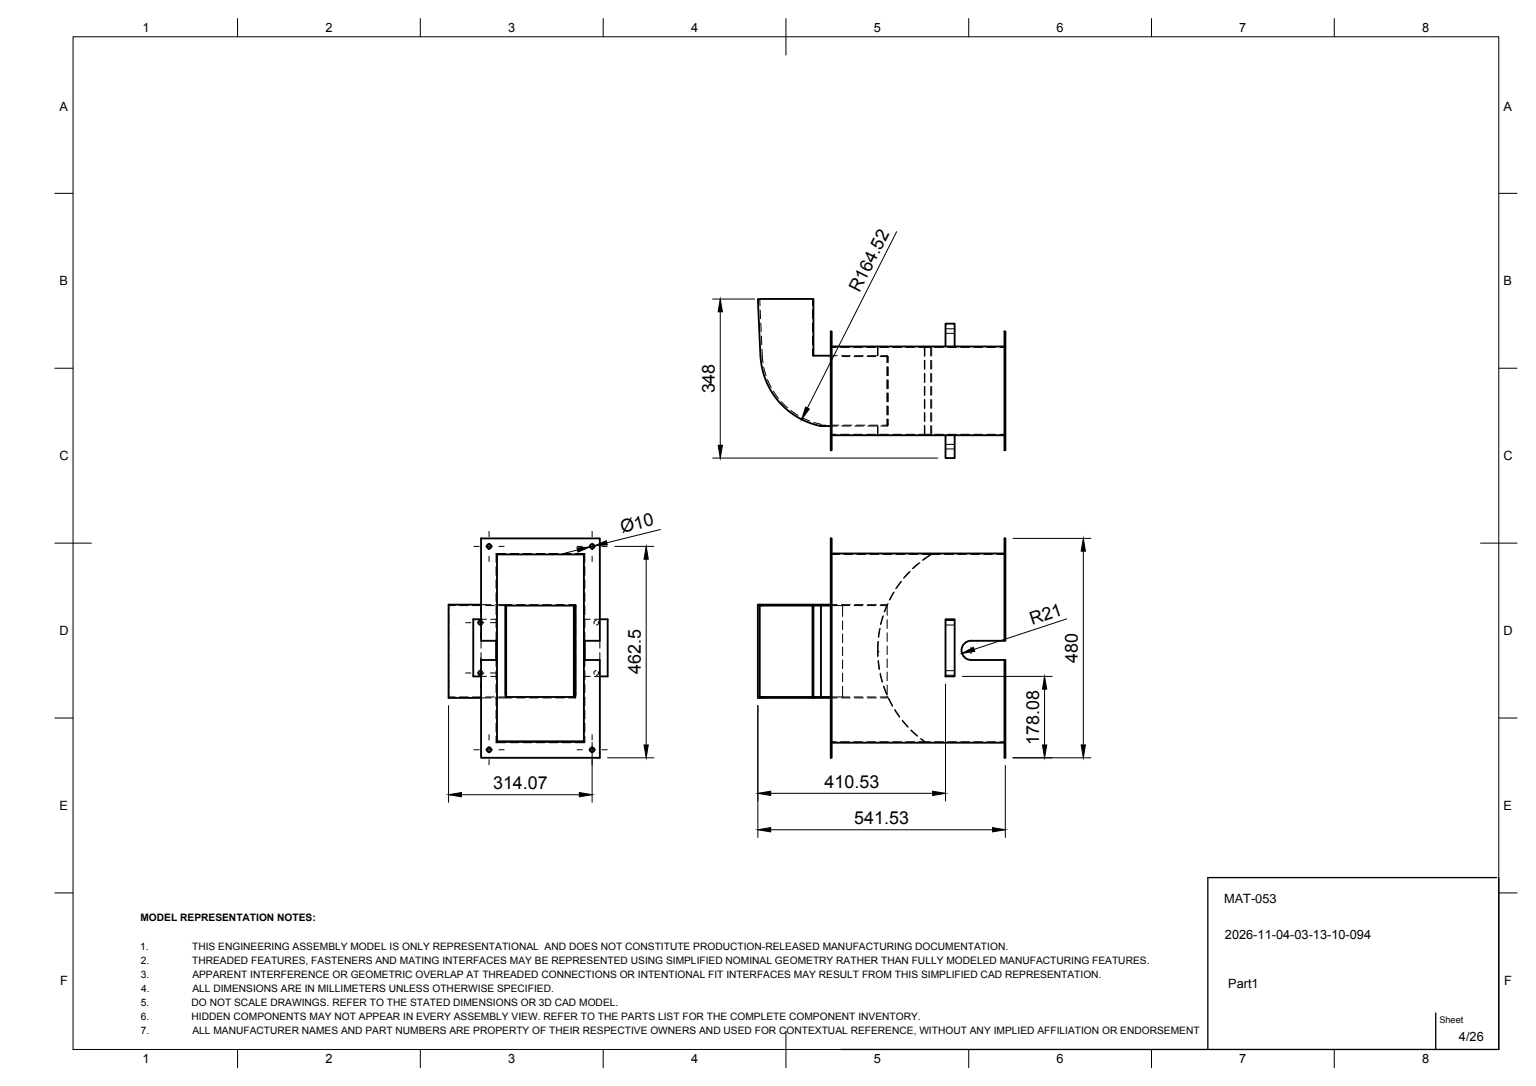
ISO-10303-21;
HEADER;
FILE_DESCRIPTION (('STEP AP214'),
    '1' );
FILE_NAME ('Part1.step',
    '2026-10-10T03:43:58',
    ( '' ),
    ( '' ),
    'SwSTEP 2.0',
    'SolidWorks 2026',
    '' );
FILE_SCHEMA (( 'AUTOMOTIVE_DESIGN' ));
ENDSEC;

DATA;
#9=VECTOR ( 'NONE', #58697, 1000.000000000000000 ) ;
#19=ORIENTED_EDGE ( 'NONE', *, *, #2654, .T. ) ;
#29=PLANE ( 'NONE',  #12068 ) ;
#34=AXIS2_PLACEMENT_3D ( 'NONE', #2299, #49415, #17054 ) ;
#77=DIRECTION ( 'NONE',  ( 1.000000000000000000, 0.000000000000000000, -0.000000000000000000 ) ) ;
#112=VECTOR ( 'NONE', #58293, 1000.000000000000000 ) ;
#116=DIRECTION ( 'NONE',  ( 0.000000000000000000, 0.000000000000000000, -1.000000000000000000 ) ) ;
#155=ORIENTED_EDGE ( 'NONE', *, *, #38259, .F. ) ;
#180=EDGE_LOOP ( 'NONE', ( #53944, #20596, #29884, #29507 ) ) ;
#185=LINE ( 'NONE', #21641, #40737 ) ;
#229=DIRECTION ( 'NONE',  ( 0.000000000000000000, 0.04541273895899431562, -0.9989683093773507050 ) ) ;
#230=EDGE_LOOP ( 'NONE', ( #67792, #13686 ) ) ;
#265=VECTOR ( 'NONE', #25443, 1000.000000000000000 ) ;
#289=ADVANCED_FACE ( 'NONE', ( #32988 ), #17141, .F. ) ;
#295=VERTEX_POINT ( 'NONE', #1681 ) ;
#297=EDGE_CURVE ( 'NONE', #67311, #11610, #65085, .T. ) ;
#314=EDGE_CURVE ( 'NONE', #536, #3478, #33702, .T. ) ;
#324=ORIENTED_EDGE ( 'NONE', *, *, #68515, .T. ) ;
#330=CARTESIAN_POINT ( 'NONE',  ( 444.9999999999999432, 225.0000000000000000, -2.000000000000000000 ) ) ;
#345=CARTESIAN_POINT ( 'NONE',  ( 0.000000000000000000, 0.000000000000000000, 380.0000000000000000 ) ) ;
#356=EDGE_CURVE ( 'NONE', #53205, #30991, #32306, .T. ) ;
#360=VECTOR ( 'NONE', #38064, 1000.000000000000000 ) ;
#401=ORIENTED_EDGE ( 'NONE', *, *, #69148, .T. ) ;
#408=ADVANCED_FACE ( 'NONE', ( #27013 ), #48440, .F. ) ;
#431=CARTESIAN_POINT ( 'NONE',  ( 111.9975424824652634, 296.0000000000000000, 529.9060149868646477 ) ) ;
#454=VERTEX_POINT ( 'NONE', #23494 ) ;
#463=EDGE_CURVE ( 'NONE', #12143, #43378, #39662, .T. ) ;
#473=EDGE_CURVE ( 'NONE', #23927, #8984, #16634, .T. ) ;
#477=ORIENTED_EDGE ( 'NONE', *, *, #56695, .T. ) ;
#491=ORIENTED_EDGE ( 'NONE', *, *, #35579, .F. ) ;
#527=DIRECTION ( 'NONE',  ( 0.000000000000000000, 0.000000000000000000, -1.000000000000000000 ) ) ;
#536=VERTEX_POINT ( 'NONE', #20279 ) ;
#575=ORIENTED_EDGE ( 'NONE', *, *, #1852, .T. ) ;
#606=VECTOR ( 'NONE', #8616, 1000.000000000000000 ) ;
#617=VECTOR ( 'NONE', #33046, 1000.000000000000000 ) ;
#626=VECTOR ( 'NONE', #27457, 1000.000000000000000 ) ;
#628=DIRECTION ( 'NONE',  ( -0.000000000000000000, -0.000000000000000000, -1.000000000000000000 ) ) ;
#653=ORIENTED_EDGE ( 'NONE', *, *, #46286, .F. ) ;
#654=EDGE_LOOP ( 'NONE', ( #13629, #60048, #33344, #59495 ) ) ;
#656=ORIENTED_EDGE ( 'NONE', *, *, #67416, .T. ) ;
#657=DIRECTION ( 'NONE',  ( 0.000000000000000000, -1.000000000000000000, 0.000000000000000000 ) ) ;
#675=DIRECTION ( 'NONE',  ( 0.000000000000000000, -1.000000000000000000, -0.000000000000000000 ) ) ;
#684=ORIENTED_EDGE ( 'NONE', *, *, #12471, .T. ) ;
#696=ORIENTED_EDGE ( 'NONE', *, *, #24415, .T. ) ;
#738=DIRECTION ( 'NONE',  ( -1.000000000000000000, 0.000000000000000000, 0.000000000000000000 ) ) ;
#821=DIRECTION ( 'NONE',  ( 0.000000000000000000, -0.000000000000000000, 1.000000000000000000 ) ) ;
#826=CYLINDRICAL_SURFACE ( 'NONE', #20311, 5.000000000000004441 ) ;
#992=LINE ( 'NONE', #5563, #37617 ) ;
#1020=EDGE_CURVE ( 'NONE', #49819, #55571, #66006, .T. ) ;
#1023=ORIENTED_EDGE ( 'NONE', *, *, #57399, .T. ) ;
#1033=CARTESIAN_POINT ( 'NONE',  ( 410.0000000000000000, -3.566368924055061292E-16, 174.3129005282752928 ) ) ;
#1037=ORIENTED_EDGE ( 'NONE', *, *, #10644, .F. ) ;
#1057=ORIENTED_EDGE ( 'NONE', *, *, #9172, .F. ) ;
#1060=FACE_OUTER_BOUND ( 'NONE', #18651, .T. ) ;
#1067=DIRECTION ( 'NONE',  ( 0.000000000000000000, 1.000000000000000000, 0.000000000000000000 ) ) ;
#1086=LINE ( 'NONE', #49961, #626 ) ;
#1118=CARTESIAN_POINT ( 'NONE',  ( 109.9975424824652634, 296.0000000000000000, 529.9060149868646477 ) ) ;
#1129=ORIENTED_EDGE ( 'NONE', *, *, #8619, .F. ) ;
#1165=DIRECTION ( 'NONE',  ( 0.000000000000000000, 0.000000000000000000, -1.000000000000000000 ) ) ;
#1188=EDGE_LOOP ( 'NONE', ( #37725, #12945, #49340, #52870, #24655, #3201, #47835, #3664 ) ) ;
#1198=VERTEX_POINT ( 'NONE', #53931 ) ;
#1228=ORIENTED_EDGE ( 'NONE', *, *, #39925, .F. ) ;
#1277=AXIS2_PLACEMENT_3D ( 'NONE', #30478, #35064, #25562 ) ;
#1357=DIRECTION ( 'NONE',  ( 0.000000000000000000, 0.000000000000000000, -1.000000000000000000 ) ) ;
#1379=DIRECTION ( 'NONE',  ( -0.000000000000000000, -0.000000000000000000, -1.000000000000000000 ) ) ;
#1399=ORIENTED_EDGE ( 'NONE', *, *, #17201, .T. ) ;
#1408=VERTEX_POINT ( 'NONE', #33562 ) ;
#1413=CARTESIAN_POINT ( 'NONE',  ( 209.9518228411288874, 0.000000000000000000, 31.43423095485942298 ) ) ;
#1424=PLANE ( 'NONE',  #7615 ) ;
#1458=DIRECTION ( 'NONE',  ( -1.000000000000000000, -0.000000000000000000, -0.000000000000000000 ) ) ;
#1464=ORIENTED_EDGE ( 'NONE', *, *, #14554, .T. ) ;
#1477=LINE ( 'NONE', #29259, #53207 ) ;
#1493=CARTESIAN_POINT ( 'NONE',  ( 410.0000000000000000, 0.000000000000000000, 380.0000000000000000 ) ) ;
#1496=ORIENTED_EDGE ( 'NONE', *, *, #11332, .F. ) ;
#1520=ORIENTED_EDGE ( 'NONE', *, *, #37790, .F. ) ;
#1535=VERTEX_POINT ( 'NONE', #23523 ) ;
#1558=EDGE_CURVE ( 'NONE', #28403, #51848, #17535, .T. ) ;
#1595=DIRECTION ( 'NONE',  ( 0.000000000000000000, 1.000000000000000000, 0.000000000000000000 ) ) ;
#1662=DIRECTION ( 'NONE',  ( -0.000000000000000000, -1.000000000000000000, -0.000000000000000000 ) ) ;
#1668=EDGE_CURVE ( 'NONE', #2382, #69500, #27304, .T. ) ;
#1680=VECTOR ( 'NONE', #34096, 1000.000000000000000 ) ;
#1681=CARTESIAN_POINT ( 'NONE',  ( 311.9975424824652350, 172.0000000000000284, 354.1673509436691347 ) ) ;
#1696=ORIENTED_EDGE ( 'NONE', *, *, #44720, .F. ) ;
#1705=ORIENTED_EDGE ( 'NONE', *, *, #28112, .T. ) ;
#1708=LINE ( 'NONE', #34768, #38008 ) ;
#1717=AXIS2_PLACEMENT_3D ( 'NONE', #66276, #45132, #30005 ) ;
#1732=CARTESIAN_POINT ( 'NONE',  ( 209.9999999999999716, 192.0000000000000000, 72.99999999999998579 ) ) ;
#1750=CARTESIAN_POINT ( 'NONE',  ( 432.4999999999999432, -18.06806526123148160, 378.0000000000000000 ) ) ;
#1783=AXIS2_PLACEMENT_3D ( 'NONE', #7114, #56339, #29267 ) ;
#1797=EDGE_LOOP ( 'NONE', ( #65731, #29293 ) ) ;
#1804=DIRECTION ( 'NONE',  ( 0.000000000000000000, -1.000000000000000000, 0.000000000000000000 ) ) ;
#1810=CARTESIAN_POINT ( 'NONE',  ( 0.000000000000000000, 190.0000000000000000, 159.3522585083728700 ) ) ;
#1812=CARTESIAN_POINT ( 'NONE',  ( 188.9999999999999432, 190.0000000000000000, 380.0000000000000000 ) ) ;
#1822=DIRECTION ( 'NONE',  ( -0.000000000000000000, -0.000000000000000000, -1.000000000000000000 ) ) ;
#1848=VECTOR ( 'NONE', #11811, 1000.000000000000000 ) ;
#1852=EDGE_CURVE ( 'NONE', #67175, #45635, #9379, .T. ) ;
#1854=CARTESIAN_POINT ( 'NONE',  ( -17.50000000000002842, -18.06806526123148160, 380.0000000000000000 ) ) ;
#1885=PLANE ( 'NONE',  #60224 ) ;
#1923=FACE_OUTER_BOUND ( 'NONE', #44162, .T. ) ;
#1974=PLANE ( 'NONE',  #39498 ) ;
#1986=LINE ( 'NONE', #30100, #9912 ) ;
#1987=CARTESIAN_POINT ( 'NONE',  ( 144.4165763529819344, -26.99999999999998224, 108.9999999999999858 ) ) ;
#2008=CARTESIAN_POINT ( 'NONE',  ( 313.9975424824652350, 172.0000000000000284, 418.0000000000000000 ) ) ;
#2012=CARTESIAN_POINT ( 'NONE',  ( 188.9999999999999432, 0.000000000000000000, 380.0000000000000000 ) ) ;
#2035=VECTOR ( 'NONE', #52358, 1000.000000000000000 ) ;
#2043=ORIENTED_EDGE ( 'NONE', *, *, #42498, .F. ) ;
#2047=CARTESIAN_POINT ( 'NONE',  ( 0.000000000000000000, 190.0000000000000000, -2.000000000000000000 ) ) ;
#2048=ORIENTED_EDGE ( 'NONE', *, *, #27631, .F. ) ;
#2063=CARTESIAN_POINT ( 'NONE',  ( 109.9975424824652634, 18.08738615523480675, 402.4289050101931480 ) ) ;
#2086=CIRCLE ( 'NONE', #66164, 246.3582898394606957 ) ;
#2097=DIRECTION ( 'NONE',  ( -1.000000000000000000, 0.000000000000000000, 0.000000000000000000 ) ) ;
#2105=ADVANCED_FACE ( 'NONE', ( #14188 ), #35648, .F. ) ;
#2115=CARTESIAN_POINT ( 'NONE',  ( 109.9975424824652634, 296.0000000000000000, 529.9060149868646477 ) ) ;
#2119=CARTESIAN_POINT ( 'NONE',  ( 309.8720357909272707, 172.0000000000000284, 536.6193948016162949 ) ) ;
#2126=VECTOR ( 'NONE', #628, 1000.000000000000000 ) ;
#2135=DIRECTION ( 'NONE',  ( 0.000000000000000000, 0.000000000000000000, 1.000000000000000000 ) ) ;
#2166=CARTESIAN_POINT ( 'NONE',  ( -12.50000000000002842, 207.5000000000000284, 378.0000000000000000 ) ) ;
#2179=DIRECTION ( 'NONE',  ( 0.000000000000000000, 0.000000000000000000, -1.000000000000000000 ) ) ;
#2210=VERTEX_POINT ( 'NONE', #64435 ) ;
#2229=AXIS2_PLACEMENT_3D ( 'NONE', #66577, #8161, #56011 ) ;
#2243=VERTEX_POINT ( 'NONE', #47217 ) ;
#2251=DIRECTION ( 'NONE',  ( 0.000000000000000000, 0.9989683093773507050, 0.04541273895899305274 ) ) ;
#2272=DIRECTION ( 'NONE',  ( 0.000000000000000000, 0.000000000000000000, 1.000000000000000000 ) ) ;
#2277=DIRECTION ( 'NONE',  ( -1.000000000000000000, 0.000000000000000000, 0.000000000000000000 ) ) ;
#2293=CARTESIAN_POINT ( 'NONE',  ( 427.4999999999999432, 207.5000000000000284, 0.000000000000000000 ) ) ;
#2299=CARTESIAN_POINT ( 'NONE',  ( 259.4165763529819060, 225.8585178651493948, 138.9999999999999716 ) ) ;
#2338=DIRECTION ( 'NONE',  ( 0.9216045519012663334, 0.000000000000000000, -0.3881301971180111110 ) ) ;
#2382=VERTEX_POINT ( 'NONE', #6028 ) ;
#2430=LINE ( 'NONE', #50964, #30805 ) ;
#2453=CARTESIAN_POINT ( 'NONE',  ( 0.000000000000000000, -2.000000000000000000, 380.0000000000000000 ) ) ;
#2507=LINE ( 'NONE', #49989, #5388 ) ;
#2535=FACE_OUTER_BOUND ( 'NONE', #48112, .T. ) ;
#2614=CARTESIAN_POINT ( 'NONE',  ( 264.4165763529819628, 225.8585178651493948, 128.9999999999999716 ) ) ;
#2626=VERTEX_POINT ( 'NONE', #43227 ) ;
#2641=AXIS2_PLACEMENT_3D ( 'NONE', #67736, #19535, #40994 ) ;
#2654=EDGE_CURVE ( 'NONE', #33368, #44925, #15052, .T. ) ;
#2674=ORIENTED_EDGE ( 'NONE', *, *, #30840, .F. ) ;
#2687=CARTESIAN_POINT ( 'NONE',  ( 111.9975424824652634, 0.000000000000000000, 256.6193948016162381 ) ) ;
#2727=ORIENTED_EDGE ( 'NONE', *, *, #23656, .F. ) ;
#2751=CARTESIAN_POINT ( 'NONE',  ( 444.9999999999999432, -35.00000000000000000, 380.0000000000000000 ) ) ;
#2809=CYLINDRICAL_SURFACE ( 'NONE', #65443, 245.3095347406802773 ) ;
#2815=DIRECTION ( 'NONE',  ( 1.000000000000000000, 0.000000000000000000, 0.000000000000000000 ) ) ;
#2816=PLANE ( 'NONE',  #19313 ) ;
#2821=DIRECTION ( 'NONE',  ( 0.000000000000000000, -1.000000000000000000, -0.000000000000000000 ) ) ;
#2831=AXIS2_PLACEMENT_3D ( 'NONE', #67732, #19884, #29741 ) ;
#2879=CARTESIAN_POINT ( 'NONE',  ( 432.4999999999999432, 207.5000000000000284, 0.000000000000000000 ) ) ;
#2887=VECTOR ( 'NONE', #14125, 1000.000000000000000 ) ;
#2902=ORIENTED_EDGE ( 'NONE', *, *, #54366, .F. ) ;
#2909=LINE ( 'NONE', #51449, #54074 ) ;
#2923=LINE ( 'NONE', #41930, #52350 ) ;
#2947=AXIS2_PLACEMENT_3D ( 'NONE', #10243, #42268, #36303 ) ;
#2957=VERTEX_POINT ( 'NONE', #32182 ) ;
#2963=LINE ( 'NONE', #57118, #66829 ) ;
#2974=DIRECTION ( 'NONE',  ( -1.000000000000000000, 0.000000000000000000, 0.000000000000000000 ) ) ;
#2986=LINE ( 'NONE', #66329, #33613 ) ;
#2999=AXIS2_PLACEMENT_3D ( 'NONE', #53087, #48837, #21109 ) ;
#3077=VECTOR ( 'NONE', #52022, 1000.000000000000000 ) ;
#3156=DIRECTION ( 'NONE',  ( -0.000000000000000000, 1.000000000000000000, -0.000000000000000000 ) ) ;
#3157=DIRECTION ( 'NONE',  ( 0.000000000000000000, 1.000000000000000000, 0.000000000000000000 ) ) ;
#3169=CARTESIAN_POINT ( 'NONE',  ( 213.7147529443549843, 172.0000000000000284, 277.7621479143228385 ) ) ;
#3182=ORIENTED_EDGE ( 'NONE', *, *, #20387, .F. ) ;
#3201=ORIENTED_EDGE ( 'NONE', *, *, #20529, .F. ) ;
#3202=DIRECTION ( 'NONE',  ( -1.000000000000000000, -0.000000000000000000, -0.000000000000000000 ) ) ;
#3213=ORIENTED_EDGE ( 'NONE', *, *, #23131, .T. ) ;
#3221=EDGE_LOOP ( 'NONE', ( #1037, #38280, #21637, #19798 ) ) ;
#3262=ORIENTED_EDGE ( 'NONE', *, *, #53398, .F. ) ;
#3263=EDGE_CURVE ( 'NONE', #46362, #11641, #10625, .T. ) ;
#3278=CARTESIAN_POINT ( 'NONE',  ( -17.50000000000002842, 207.5000000000000284, 380.0000000000000000 ) ) ;
#3313=LINE ( 'NONE', #24774, #4136 ) ;
#3315=ORIENTED_EDGE ( 'NONE', *, *, #43959, .F. ) ;
#3333=EDGE_CURVE ( 'NONE', #9171, #11778, #44252, .T. ) ;
#3363=FACE_OUTER_BOUND ( 'NONE', #61772, .T. ) ;
#3375=LINE ( 'NONE', #67747, #44396 ) ;
#3403=ORIENTED_EDGE ( 'NONE', *, *, #15348, .F. ) ;
#3425=DIRECTION ( 'NONE',  ( -0.8532989592251508659, 0.000000000000000000, 0.5214219847544543374 ) ) ;
#3463=CARTESIAN_POINT ( 'NONE',  ( 422.4999999999999432, 207.5000000000000284, -2.000000000000000000 ) ) ;
#3478=VERTEX_POINT ( 'NONE', #65860 ) ;
#3486=CARTESIAN_POINT ( 'NONE',  ( 209.9518228411288874, 18.00000000000002842, 31.43423095485942298 ) ) ;
#3498=EDGE_CURVE ( 'NONE', #14375, #1535, #61261, .T. ) ;
#3500=CARTESIAN_POINT ( 'NONE',  ( 149.4165763529819344, -26.99999999999998224, 108.9999999999999858 ) ) ;
#3521=CARTESIAN_POINT ( 'NONE',  ( -12.50000000000002842, -18.06806526123148160, 380.0000000000000000 ) ) ;
#3574=DIRECTION ( 'NONE',  ( 1.000000000000000000, 0.000000000000000000, -0.000000000000000000 ) ) ;
#3602=CARTESIAN_POINT ( 'NONE',  ( 427.4999999999999432, -18.06806526123148160, -2.000000000000000000 ) ) ;
#3604=DIRECTION ( 'NONE',  ( 2.220446049250313081E-16, 0.000000000000000000, 1.000000000000000000 ) ) ;
#3610=CYLINDRICAL_SURFACE ( 'NONE', #28683, 246.3582898394606957 ) ;
#3619=CARTESIAN_POINT ( 'NONE',  ( 444.9999999999999432, 225.0000000000000000, 0.000000000000000000 ) ) ;
#3653=FACE_BOUND ( 'NONE', #46999, .T. ) ;
#3654=DIRECTION ( 'NONE',  ( -1.000000000000000000, 0.000000000000000000, 0.000000000000000000 ) ) ;
#3659=ORIENTED_EDGE ( 'NONE', *, *, #14979, .F. ) ;
#3664=ORIENTED_EDGE ( 'NONE', *, *, #5871, .F. ) ;
#3673=( LENGTH_UNIT ( ) NAMED_UNIT ( * ) SI_UNIT ( .MILLI., .METRE. ) );
#3696=FACE_OUTER_BOUND ( 'NONE', #32892, .T. ) ;
#3707=ORIENTED_EDGE ( 'NONE', *, *, #60071, .F. ) ;
#3743=CARTESIAN_POINT ( 'NONE',  ( 149.4165763529819344, 225.8585178651493663, 108.9999999999999858 ) ) ;
#3750=DIRECTION ( 'NONE',  ( -1.000000000000000000, 0.000000000000000000, 0.000000000000000000 ) ) ;
#3790=EDGE_LOOP ( 'NONE', ( #19909, #52215, #66218, #50084 ) ) ;
#3813=EDGE_CURVE ( 'NONE', #2957, #57714, #49733, .T. ) ;
#3841=FACE_OUTER_BOUND ( 'NONE', #20050, .T. ) ;
#3843=EDGE_CURVE ( 'NONE', #35195, #22151, #28650, .T. ) ;
#3853=DIRECTION ( 'NONE',  ( -1.000000000000000000, 0.000000000000000000, 0.000000000000000000 ) ) ;
#3862=CYLINDRICAL_SURFACE ( 'NONE', #39982, 5.000000000000000888 ) ;
#3869=LINE ( 'NONE', #20730, #10810 ) ;
#3895=AXIS2_PLACEMENT_3D ( 'NONE', #1732, #33745, #7004 ) ;
#3933=VECTOR ( 'NONE', #53497, 1000.000000000000000 ) ;
#3945=LINE ( 'NONE', #57754, #60605 ) ;
#3947=CARTESIAN_POINT ( 'NONE',  ( 444.9999999999999432, -35.00000000000000000, -2.000000000000000000 ) ) ;
#3950=PRODUCT_DEFINITION ( 'UNKNOWN', '', #68169, #43669 ) ;
#3953=DIRECTION ( 'NONE',  ( 0.000000000000000000, 0.000000000000000000, -1.000000000000000000 ) ) ;
#3979=EDGE_LOOP ( 'NONE', ( #60158, #1057, #656, #3707 ) ) ;
#3987=AXIS2_PLACEMENT_3D ( 'NONE', #45053, #29926, #14093 ) ;
#3989=CYLINDRICAL_SURFACE ( 'NONE', #60363, 246.3582898394606957 ) ;
#4006=DIRECTION ( 'NONE',  ( -0.000000000000000000, -0.000000000000000000, 1.000000000000000000 ) ) ;
#4015=CARTESIAN_POINT ( 'NONE',  ( 444.9999999999999432, 225.0000000000000000, 380.0000000000000000 ) ) ;
#4018=FACE_BOUND ( 'NONE', #5277, .T. ) ;
#4026=SURFACE_SIDE_STYLE ('',( #64140 ) ) ;
#4032=DIRECTION ( 'NONE',  ( -0.000000000000000000, 1.000000000000000000, 0.000000000000000000 ) ) ;
#4136=VECTOR ( 'NONE', #3654, 1000.000000000000000 ) ;
#4195=EDGE_CURVE ( 'NONE', #14640, #7559, #37718, .T. ) ;
#4205=ORIENTED_EDGE ( 'NONE', *, *, #66591, .T. ) ;
#4227=CARTESIAN_POINT ( 'NONE',  ( 230.9999999999999432, -2.000000000000000000, 0.000000000000000000 ) ) ;
#4247=ORIENTED_EDGE ( 'NONE', *, *, #45253, .T. ) ;
#4253=VECTOR ( 'NONE', #53682, 1000.000000000000000 ) ;
#4264=LINE ( 'NONE', #35927, #67110 ) ;
#4296=DIRECTION ( 'NONE',  ( 0.000000000000000000, 0.000000000000000000, 1.000000000000000000 ) ) ;
#4321=ADVANCED_FACE ( 'NONE', ( #52442, #69302, #10552 ), #59082, .F. ) ;
#4333=DIRECTION ( 'NONE',  ( 0.000000000000000000, -0.000000000000000000, 1.000000000000000000 ) ) ;
#4372=EDGE_CURVE ( 'NONE', #11778, #9171, #17235, .T. ) ;
#4381=CARTESIAN_POINT ( 'NONE',  ( 230.9999999999999432, 225.0000000000000000, -2.000000000000000000 ) ) ;
#4410=AXIS2_PLACEMENT_3D ( 'NONE', #23079, #24730, #27991 ) ;
#4431=EDGE_LOOP ( 'NONE', ( #49238, #30176, #26418, #57787, #61721, #36911, #47133, #38510 ) ) ;
#4435=CARTESIAN_POINT ( 'NONE',  ( 209.3223706822284100, 18.00000000000002842, 31.44247402469554942 ) ) ;
#4438=ORIENTED_EDGE ( 'NONE', *, *, #56470, .T. ) ;
#4439=EDGE_CURVE ( 'NONE', #61512, #35195, #55470, .T. ) ;
#4442=CARTESIAN_POINT ( 'NONE',  ( 144.4165763529819344, -26.99999999999998224, 129.0000000000000000 ) ) ;
#4445=AXIS2_PLACEMENT_3D ( 'NONE', #32054, #54172, #26777 ) ;
#4461=ORIENTED_EDGE ( 'NONE', *, *, #65946, .F. ) ;
#4514=EDGE_LOOP ( 'NONE', ( #56246, #66798, #21095, #54977 ) ) ;
#4522=VERTEX_POINT ( 'NONE', #37906 ) ;
#4527=EDGE_CURVE ( 'NONE', #58159, #37433, #21720, .T. ) ;
#4540=AXIS2_PLACEMENT_3D ( 'NONE', #13314, #56207, #63225 ) ;
#4549=CARTESIAN_POINT ( 'NONE',  ( 422.4999999999999432, 207.5000000000000284, 378.0000000000000000 ) ) ;
#4559=CARTESIAN_POINT ( 'NONE',  ( 188.9999999999999432, 192.0000000000000000, 380.0000000000000000 ) ) ;
#4573=ORIENTED_EDGE ( 'NONE', *, *, #57997, .F. ) ;
#4597=VERTEX_POINT ( 'NONE', #11501 ) ;
#4647=ORIENTED_EDGE ( 'NONE', *, *, #18931, .F. ) ;
#4665=DIRECTION ( 'NONE',  ( -0.000000000000000000, -1.000000000000000000, -0.000000000000000000 ) ) ;
#4690=AXIS2_PLACEMENT_3D ( 'NONE', #10679, #63473, #25852 ) ;
#4716=ORIENTED_EDGE ( 'NONE', *, *, #57128, .F. ) ;
#4717=ORIENTED_EDGE ( 'NONE', *, *, #37321, .T. ) ;
#4729=PLANE ( 'NONE',  #13598 ) ;
#4777=FACE_BOUND ( 'NONE', #67741, .T. ) ;
#4797=ORIENTED_EDGE ( 'NONE', *, *, #48258, .F. ) ;
#4803=CARTESIAN_POINT ( 'NONE',  ( 311.9975424824652350, 0.000000000000000000, 254.5114349394235091 ) ) ;
#4874=DIRECTION ( 'NONE',  ( 0.000000000000000000, -1.000000000000000000, 0.000000000000000000 ) ) ;
#4875=AXIS2_PLACEMENT_3D ( 'NONE', #67150, #56217, #8033 ) ;
#4894=ORIENTED_EDGE ( 'NONE', *, *, #26906, .F. ) ;
#4899=DIRECTION ( 'NONE',  ( 0.01527021686369653929, 0.000000000000000000, 0.9998834034410890581 ) ) ;
#4947=CARTESIAN_POINT ( 'NONE',  ( -2.000000000000000000, 192.0000000000000000, 0.000000000000000000 ) ) ;
#4950=CARTESIAN_POINT ( 'NONE',  ( 0.000000000000000000, 190.0000000000000000, 380.0000000000000000 ) ) ;
#4992=ORIENTED_EDGE ( 'NONE', *, *, #9172, .T. ) ;
#4993=DIRECTION ( 'NONE',  ( 0.000000000000000000, -0.04541273895899431562, 0.9989683093773507050 ) ) ;
#5038=DIRECTION ( 'NONE',  ( -0.000000000000000000, 1.000000000000000000, -0.000000000000000000 ) ) ;
#5058=ORIENTED_EDGE ( 'NONE', *, *, #48308, .F. ) ;
#5062=FACE_OUTER_BOUND ( 'NONE', #58838, .T. ) ;
#5083=ORIENTED_EDGE ( 'NONE', *, *, #5149, .F. ) ;
#5090=ADVANCED_FACE ( 'NONE', ( #7034 ), #16879, .T. ) ;
#5130=EDGE_LOOP ( 'NONE', ( #32465, #36018, #4205, #43467 ) ) ;
#5133=VERTEX_POINT ( 'NONE', #56967 ) ;
#5149=EDGE_CURVE ( 'NONE', #9638, #32243, #67191, .T. ) ;
#5170=VERTEX_POINT ( 'NONE', #57308 ) ;
#5173=VECTOR ( 'NONE', #39093, 1000.000000000000000 ) ;
#5206=VERTEX_POINT ( 'NONE', #51345 ) ;
#5219=VECTOR ( 'NONE', #53760, 1000.000000000000000 ) ;
#5221=ADVANCED_FACE ( 'NONE', ( #3841 ), #18979, .T. ) ;
#5246=DIRECTION ( 'NONE',  ( 1.000000000000000000, 0.000000000000000000, 0.000000000000000000 ) ) ;
#5273=VECTOR ( 'NONE', #19989, 1000.000000000000000 ) ;
#5277=EDGE_LOOP ( 'NONE', ( #54537, #58069 ) ) ;
#5289=AXIS2_PLACEMENT_3D ( 'NONE', #24118, #66692, #13218 ) ;
#5291=VERTEX_POINT ( 'NONE', #61545 ) ;
#5326=ORIENTED_EDGE ( 'NONE', *, *, #12858, .F. ) ;
#5334=VECTOR ( 'NONE', #56402, 1000.000000000000000 ) ;
#5360=FACE_OUTER_BOUND ( 'NONE', #36717, .T. ) ;
#5368=DIRECTION ( 'NONE',  ( 0.000000000000000000, 0.9997420440737085912, 0.02271222823333339524 ) ) ;
#5388=VECTOR ( 'NONE', #1458, 1000.000000000000000 ) ;
#5406=CARTESIAN_POINT ( 'NONE',  ( 149.4165763529819344, 225.8585178651493663, 138.9999999999999716 ) ) ;
#5435=VERTEX_POINT ( 'NONE', #48109 ) ;
#5460=VERTEX_POINT ( 'NONE', #31954 ) ;
#5468=ORIENTED_EDGE ( 'NONE', *, *, #11176, .F. ) ;
#5471=AXIS2_PLACEMENT_3D ( 'NONE', #2293, #57141, #30065 ) ;
#5499=EDGE_LOOP ( 'NONE', ( #1520, #5685, #65376, #32229 ) ) ;
#5521=CARTESIAN_POINT ( 'NONE',  ( 188.9999999999999432, -57.00000000000007816, 72.99999999999998579 ) ) ;
#5522=VECTOR ( 'NONE', #44921, 1000.000000000000000 ) ;
#5554=CARTESIAN_POINT ( 'NONE',  ( 209.9518228411288874, 0.000000000000000000, 31.43423095485942298 ) ) ;
#5563=CARTESIAN_POINT ( 'NONE',  ( 0.000000000000000000, 0.000000000000000000, 161.3522585083728700 ) ) ;
#5634=ADVANCED_FACE ( 'NONE', ( #18897, #62505, #55840 ), #7660, .T. ) ;
#5685=ORIENTED_EDGE ( 'NONE', *, *, #46043, .F. ) ;
#5728=CARTESIAN_POINT ( 'NONE',  ( -22.50000000000003197, 207.5000000000000284, 0.000000000000000000 ) ) ;
#5755=ORIENTED_EDGE ( 'NONE', *, *, #6077, .F. ) ;
#5770=EDGE_CURVE ( 'NONE', #4597, #14754, #14650, .T. ) ;
#5771=LINE ( 'NONE', #58542, #12839 ) ;
#5773=EDGE_CURVE ( 'NONE', #295, #34394, #69137, .T. ) ;
#5805=CYLINDRICAL_SURFACE ( 'NONE', #5471, 5.000000000000004441 ) ;
#5814=ORIENTED_EDGE ( 'NONE', *, *, #59443, .T. ) ;
#5815=ORIENTED_EDGE ( 'NONE', *, *, #50680, .T. ) ;
#5830=VECTOR ( 'NONE', #23562, 1000.000000000000000 ) ;
#5832=LINE ( 'NONE', #27288, #40983 ) ;
#5838=AXIS2_PLACEMENT_3D ( 'NONE', #65367, #38269, #54083 ) ;
#5865=CARTESIAN_POINT ( 'NONE',  ( 422.4999999999999432, 207.5000000000000284, 0.000000000000000000 ) ) ;
#5871=EDGE_CURVE ( 'NONE', #8192, #55258, #21304, .T. ) ;
#5913=VECTOR ( 'NONE', #66847, 1000.000000000000000 ) ;
#5921=CARTESIAN_POINT ( 'NONE',  ( -17.50000000000002842, 207.5000000000000284, 378.0000000000000000 ) ) ;
#5927=EDGE_LOOP ( 'NONE', ( #13537, #18254, #49283, #3262 ) ) ;
#5955=EDGE_CURVE ( 'NONE', #18015, #1535, #16375, .T. ) ;
#5995=FACE_OUTER_BOUND ( 'NONE', #41690, .T. ) ;
#6028=CARTESIAN_POINT ( 'NONE',  ( 444.9999999999999432, -35.00000000000000000, -2.000000000000000000 ) ) ;
#6030=CIRCLE ( 'NONE', #53220, 246.3582898394606957 ) ;
#6043=CARTESIAN_POINT ( 'NONE',  ( 0.000000000000000000, 172.0000000000000284, 0.000000000000000000 ) ) ;
#6060=PLANE ( 'NONE',  #27073 ) ;
#6061=ORIENTED_EDGE ( 'NONE', *, *, #12416, .T. ) ;
#6077=EDGE_CURVE ( 'NONE', #61540, #31482, #44849, .T. ) ;
#6083=DIRECTION ( 'NONE',  ( 0.000000000000000000, 1.000000000000000000, -0.000000000000000000 ) ) ;
#6106=DIRECTION ( 'NONE',  ( -0.000000000000000000, -0.000000000000000000, -1.000000000000000000 ) ) ;
#6108=DIRECTION ( 'NONE',  ( 0.000000000000000000, 0.000000000000000000, -1.000000000000000000 ) ) ;
#6122=ORIENTED_EDGE ( 'NONE', *, *, #52932, .F. ) ;
#6133=CARTESIAN_POINT ( 'NONE',  ( 109.9975424824652634, 295.8720703627916464, 535.5371946177799600 ) ) ;
#6138=CARTESIAN_POINT ( 'NONE',  ( 209.3223706822284100, 190.0000000000000000, 31.44247402469554942 ) ) ;
#6140=FACE_OUTER_BOUND ( 'NONE', #41466, .T. ) ;
#6151=DIRECTION ( 'NONE',  ( -0.000000000000000000, 0.9989683093773507050, 0.04541273895899431562 ) ) ;
#6159=EDGE_CURVE ( 'NONE', #61576, #36681, #9645, .T. ) ;
#6164=CARTESIAN_POINT ( 'NONE',  ( -35.00000000000002842, -35.00000000000000000, 378.0000000000000000 ) ) ;
#6206=EDGE_LOOP ( 'NONE', ( #52112, #47625, #22210, #62990 ) ) ;
#6228=LINE ( 'NONE', #12562, #10461 ) ;
#6232=ORIENTED_EDGE ( 'NONE', *, *, #63129, .F. ) ;
#6244=DIRECTION ( 'NONE',  ( 0.000000000000000000, -0.000000000000000000, -1.000000000000000000 ) ) ;
#6255=DIRECTION ( 'NONE',  ( 1.000000000000000000, 0.000000000000000000, -2.220446049250313081E-16 ) ) ;
#6291=CARTESIAN_POINT ( 'NONE',  ( 209.3223706822284100, 172.0000000000000284, 31.44247402469554942 ) ) ;
#6337=FACE_OUTER_BOUND ( 'NONE', #63369, .T. ) ;
#6380=DIRECTION ( 'NONE',  ( 0.000000000000000000, 1.000000000000000000, 0.000000000000000000 ) ) ;
#6383=LINE ( 'NONE', #66198, #11852 ) ;
#6421=AXIS2_PLACEMENT_3D ( 'NONE', #57042, #65428, #64729 ) ;
#6431=CARTESIAN_POINT ( 'NONE',  ( 0.000000000000000000, 190.0000000000000000, 380.0000000000000000 ) ) ;
#6490=COLOUR_RGB ( '',0.7921568627450980005, 0.8196078431372548767, 0.9333333333333333481 ) ;
#6535=ORIENTED_EDGE ( 'NONE', *, *, #1558, .F. ) ;
#6549=DIRECTION ( 'NONE',  ( -0.000000000000000000, -0.000000000000000000, -1.000000000000000000 ) ) ;
#6561=EDGE_LOOP ( 'NONE', ( #54504, #19764, #6061, #47746 ) ) ;
#6566=CARTESIAN_POINT ( 'NONE',  ( 141.9165763529819344, -52.00000000000000711, 108.9999999999999858 ) ) ;
#6598=ADVANCED_FACE ( 'NONE', ( #19914 ), #68769, .T. ) ;
#6608=DIRECTION ( 'NONE',  ( -0.000000000000000000, -0.000000000000000000, 1.000000000000000000 ) ) ;
#6634=CARTESIAN_POINT ( 'NONE',  ( 141.9165763529819344, -52.00000000000000711, 108.9999999999999858 ) ) ;
#6639=CARTESIAN_POINT ( 'NONE',  ( 307.2575771313985342, 20.00000000000003197, 256.6193948016162381 ) ) ;
#6649=DIRECTION ( 'NONE',  ( -0.000000000000000000, -0.000000000000000000, -1.000000000000000000 ) ) ;
#6679=AXIS2_PLACEMENT_3D ( 'NONE', #31791, #27540, #16640 ) ;
#6691=CARTESIAN_POINT ( 'NONE',  ( 432.4999999999999432, -18.06806526123148160, -2.000000000000000000 ) ) ;
#6761=CARTESIAN_POINT ( 'NONE',  ( 309.8720357909272707, 0.000000000000000000, 256.6193948016162381 ) ) ;
#6764=AXIS2_PLACEMENT_3D ( 'NONE', #9599, #31061, #56396 ) ;
#6812=CARTESIAN_POINT ( 'NONE',  ( 0.000000000000000000, -52.00000000000000711, 0.000000000000000000 ) ) ;
#6841=ORIENTED_EDGE ( 'NONE', *, *, #46881, .T. ) ;
#6954=ORIENTED_EDGE ( 'NONE', *, *, #54151, .F. ) ;
#6980=PLANE ( 'NONE',  #36971 ) ;
#7004=DIRECTION ( 'NONE',  ( 0.000000000000000000, 0.000000000000000000, -1.000000000000000000 ) ) ;
#7026=ORIENTED_EDGE ( 'NONE', *, *, #34004, .T. ) ;
#7034=FACE_OUTER_BOUND ( 'NONE', #25684, .T. ) ;
#7037=DIRECTION ( 'NONE',  ( -0.000000000000000000, 1.000000000000000000, -0.000000000000000000 ) ) ;
#7038=ORIENTED_EDGE ( 'NONE', *, *, #66322, .T. ) ;
#7088=EDGE_LOOP ( 'NONE', ( #22506, #12483, #32040, #52088 ) ) ;
#7114=CARTESIAN_POINT ( 'NONE',  ( 427.4999999999999432, -18.06806526123148160, 0.000000000000000000 ) ) ;
#7118=ORIENTED_EDGE ( 'NONE', *, *, #12947, .F. ) ;
#7123=ORIENTED_EDGE ( 'NONE', *, *, #20168, .F. ) ;
#7154=VECTOR ( 'NONE', #61070, 1000.000000000000000 ) ;
#7194=VECTOR ( 'NONE', #13454, 1000.000000000000000 ) ;
#7251=DIRECTION ( 'NONE',  ( -0.000000000000000000, -0.000000000000000000, -1.000000000000000000 ) ) ;
#7254=EDGE_CURVE ( 'NONE', #2382, #10473, #24021, .T. ) ;
#7257=VECTOR ( 'NONE', #66815, 1000.000000000000000 ) ;
#7329=CARTESIAN_POINT ( 'NONE',  ( 209.3223706822284100, 0.000000000000000000, 277.8007638641562380 ) ) ;
#7336=EDGE_CURVE ( 'NONE', #55844, #22362, #1086, .T. ) ;
#7345=VERTEX_POINT ( 'NONE', #65106 ) ;
#7396=CYLINDRICAL_SURFACE ( 'NONE', #22759, 21.00000000000000355 ) ;
#7447=CARTESIAN_POINT ( 'NONE',  ( 266.9165763529819628, 242.0000000000000000, 108.9999999999999858 ) ) ;
#7497=DIRECTION ( 'NONE',  ( 1.000000000000000000, -0.000000000000000000, 0.000000000000000000 ) ) ;
#7509=DIRECTION ( 'NONE',  ( 1.000000000000000000, 0.000000000000000000, 0.000000000000000000 ) ) ;
#7559=VERTEX_POINT ( 'NONE', #34335 ) ;
#7578=EDGE_CURVE ( 'NONE', #28503, #49819, #29809, .T. ) ;
#7592=EDGE_LOOP ( 'NONE', ( #55217, #67911, #28990, #60492 ) ) ;
#7606=ORIENTED_EDGE ( 'NONE', *, *, #43316, .T. ) ;
#7615=AXIS2_PLACEMENT_3D ( 'NONE', #17959, #33788, #11978 ) ;
#7622=DIRECTION ( 'NONE',  ( 0.3881301971180111110, 0.000000000000000000, 0.9216045519012663334 ) ) ;
#7652=CARTESIAN_POINT ( 'NONE',  ( -35.00000000000002842, -35.00000000000000000, -2.000000000000000000 ) ) ;
#7657=ORIENTED_EDGE ( 'NONE', *, *, #40365, .F. ) ;
#7660=PLANE ( 'NONE',  #62237 ) ;
#7665=ORIENTED_EDGE ( 'NONE', *, *, #18623, .T. ) ;
#7675=CARTESIAN_POINT ( 'NONE',  ( 209.9518228411288874, -1.426547569622074412E-15, 31.43423095485942298 ) ) ;
#7688=DIRECTION ( 'NONE',  ( 0.000000000000000000, 1.000000000000000000, 0.000000000000000000 ) ) ;
#7702=LINE ( 'NONE', #28809, #8561 ) ;
#7754=DIRECTION ( 'NONE',  ( -0.000000000000000000, 0.000000000000000000, -1.000000000000000000 ) ) ;
#7765=ORIENTED_EDGE ( 'NONE', *, *, #14723, .T. ) ;
#7782=CARTESIAN_POINT ( 'NONE',  ( 311.9975424824652350, 179.2896996249788799, 369.5505932007772003 ) ) ;
#7832=EDGE_LOOP ( 'NONE', ( #653, #10988, #66625, #15834 ) ) ;
#7837=VERTEX_POINT ( 'NONE', #39516 ) ;
#7838=FACE_OUTER_BOUND ( 'NONE', #5130, .T. ) ;
#7891=CARTESIAN_POINT ( 'NONE',  ( 209.9999999999999716, -57.00000000000007816, 72.99999999999998579 ) ) ;
#7902=CIRCLE ( 'NONE', #51730, 5.000000000000000888 ) ;
#7911=LINE ( 'NONE', #18466, #44802 ) ;
#7913=DIRECTION ( 'NONE',  ( 1.000000000000000000, 0.000000000000000000, -0.000000000000000000 ) ) ;
#7936=CARTESIAN_POINT ( 'NONE',  ( 209.9518228411288874, 170.0000000000000284, 31.43423095485942298 ) ) ;
#7965=DIRECTION ( 'NONE',  ( -0.000000000000000000, -1.000000000000000000, -0.000000000000000000 ) ) ;
#8005=CIRCLE ( 'NONE', #25993, 246.3582898394606957 ) ;
#8031=ORIENTED_EDGE ( 'NONE', *, *, #32572, .T. ) ;
#8033=DIRECTION ( 'NONE',  ( 0.000000000000000000, 0.000000000000000000, 1.000000000000000000 ) ) ;
#8036=EDGE_CURVE ( 'NONE', #41448, #36497, #2923, .T. ) ;
#8088=LINE ( 'NONE', #14058, #18215 ) ;
#8110=VECTOR ( 'NONE', #48451, 1000.000000000000000 ) ;
#8161=DIRECTION ( 'NONE',  ( -0.000000000000000000, -0.000000000000000000, -1.000000000000000000 ) ) ;
#8163=VERTEX_POINT ( 'NONE', #1810 ) ;
#8192=VERTEX_POINT ( 'NONE', #4227 ) ;
#8203=ORIENTED_EDGE ( 'NONE', *, *, #37152, .T. ) ;
#8210=CARTESIAN_POINT ( 'NONE',  ( 259.4165763529819060, -27.00000000000000355, 108.9999999999999858 ) ) ;
#8215=VECTOR ( 'NONE', #13644, 1000.000000000000000 ) ;
#8222=CIRCLE ( 'NONE', #47503, 5.000000000000004441 ) ;
#8258=DIRECTION ( 'NONE',  ( 0.000000000000000000, 0.000000000000000000, -1.000000000000000000 ) ) ;
#8261=CIRCLE ( 'NONE', #62168, 245.3095347406802205 ) ;
#8279=EDGE_LOOP ( 'NONE', ( #41736, #58624, #62946, #38975 ) ) ;
#8284=PLANE ( 'NONE',  #64935 ) ;
#8319=DIRECTION ( 'NONE',  ( 1.000000000000000000, 0.000000000000000000, 0.000000000000000000 ) ) ;
#8357=VERTEX_POINT ( 'NONE', #63316 ) ;
#8365=DIRECTION ( 'NONE',  ( 0.000000000000000000, 0.000000000000000000, 1.000000000000000000 ) ) ;
#8367=VECTOR ( 'NONE', #8404, 1000.000000000000114 ) ;
#8394=CARTESIAN_POINT ( 'NONE',  ( 188.9999999999999432, -0.000000000000000000, 0.000000000000000000 ) ) ;
#8404=DIRECTION ( 'NONE',  ( 0.9216045519012663334, 7.132737848110168930E-16, -0.3881301971180111110 ) ) ;
#8410=VECTOR ( 'NONE', #8721, 1000.000000000000000 ) ;
#8434=ORIENTED_EDGE ( 'NONE', *, *, #19290, .F. ) ;
#8461=LINE ( 'NONE', #29913, #12935 ) ;
#8560=CARTESIAN_POINT ( 'NONE',  ( 109.9975424824652634, 18.08738615523480675, 402.4289050101931480 ) ) ;
#8561=VECTOR ( 'NONE', #19278, 1000.000000000000000 ) ;
#8569=EDGE_CURVE ( 'NONE', #52352, #61540, #36844, .T. ) ;
#8578=VECTOR ( 'NONE', #229, 1000.000000000000114 ) ;
#8579=CARTESIAN_POINT ( 'NONE',  ( 188.9999999999999432, -57.00000000000007816, -2.000000000000000888 ) ) ;
#8603=VERTEX_POINT ( 'NONE', #27306 ) ;
#8606=VECTOR ( 'NONE', #57939, 1000.000000000000000 ) ;
#8616=DIRECTION ( 'NONE',  ( 1.000000000000000000, 0.000000000000000000, 0.000000000000000000 ) ) ;
#8619=EDGE_CURVE ( 'NONE', #47553, #69411, #23095, .T. ) ;
#8635=FACE_BOUND ( 'NONE', #38514, .T. ) ;
#8654=ORIENTED_EDGE ( 'NONE', *, *, #66322, .F. ) ;
#8665=CIRCLE ( 'NONE', #18797, 160.5210298272983209 ) ;
#8695=ORIENTED_EDGE ( 'NONE', *, *, #69243, .F. ) ;
#8701=CARTESIAN_POINT ( 'NONE',  ( 209.3223706822284100, 190.0000000000000000, 277.8007638641562380 ) ) ;
#8721=DIRECTION ( 'NONE',  ( 1.000000000000000000, 0.000000000000000000, -2.220446049250313081E-16 ) ) ;
#8753=AXIS2_PLACEMENT_3D ( 'NONE', #56796, #56097, #7913 ) ;
#8794=ORIENTED_EDGE ( 'NONE', *, *, #38584, .T. ) ;
#8837=ORIENTED_EDGE ( 'NONE', *, *, #39272, .T. ) ;
#8871=ORIENTED_EDGE ( 'NONE', *, *, #4195, .T. ) ;
#8903=AXIS2_PLACEMENT_3D ( 'NONE', #51006, #2815, #24279 ) ;
#8940=FACE_BOUND ( 'NONE', #15808, .T. ) ;
#8958=CIRCLE ( 'NONE', #24679, 246.3582898394606957 ) ;
#8984=VERTEX_POINT ( 'NONE', #30283 ) ;
#9048=ADVANCED_FACE ( 'NONE', ( #9864 ), #27052, .F. ) ;
#9077=ORIENTED_EDGE ( 'NONE', *, *, #25580, .F. ) ;
#9114=LINE ( 'NONE', #30572, #3077 ) ;
#9119=AXIS2_PLACEMENT_3D ( 'NONE', #29665, #68005, #56749 ) ;
#9143=EDGE_CURVE ( 'NONE', #8163, #57196, #39709, .T. ) ;
#9144=CARTESIAN_POINT ( 'NONE',  ( 266.9165763529819628, 192.0000000000000000, 108.9999999999999858 ) ) ;
#9171=VERTEX_POINT ( 'NONE', #60804 ) ;
#9172=EDGE_CURVE ( 'NONE', #15171, #33294, #65400, .T. ) ;
#9181=VERTEX_POINT ( 'NONE', #28814 ) ;
#9209=AXIS2_PLACEMENT_3D ( 'NONE', #58153, #69031, #20862 ) ;
#9210=ORIENTED_EDGE ( 'NONE', *, *, #25346, .T. ) ;
#9214=ORIENTED_EDGE ( 'NONE', *, *, #23752, .T. ) ;
#9222=DIRECTION ( 'NONE',  ( 0.000000000000000000, 1.000000000000000000, 0.000000000000000000 ) ) ;
#9248=LINE ( 'NONE', #3619, #40081 ) ;
#9286=FACE_OUTER_BOUND ( 'NONE', #58448, .T. ) ;
#9289=CARTESIAN_POINT ( 'NONE',  ( 427.4999999999999432, -18.06806526123148160, -2.000000000000000000 ) ) ;
#9309=VECTOR ( 'NONE', #39059, 1000.000000000000000 ) ;
#9322=ORIENTED_EDGE ( 'NONE', *, *, #36064, .F. ) ;
#9349=DIRECTION ( 'NONE',  ( -1.000000000000000000, 0.000000000000000000, 0.000000000000000000 ) ) ;
#9379=CIRCLE ( 'NONE', #62143, 5.000000000000000888 ) ;
#9386=EDGE_LOOP ( 'NONE', ( #23868, #37434, #5468, #46800 ) ) ;
#9404=DIRECTION ( 'NONE',  ( 0.000000000000000000, 1.000000000000000000, -0.000000000000000000 ) ) ;
#9418=AXIS2_PLACEMENT_3D ( 'NONE', #36587, #15474, #68257 ) ;
#9427=DIRECTION ( 'NONE',  ( -1.000000000000000000, 0.000000000000000000, 0.000000000000000000 ) ) ;
#9439=DIRECTION ( 'NONE',  ( -1.000000000000000000, 0.000000000000000000, 0.000000000000000000 ) ) ;
#9486=CARTESIAN_POINT ( 'NONE',  ( 444.9999999999999432, 225.0000000000000000, -2.000000000000000000 ) ) ;
#9518=VECTOR ( 'NONE', #48761, 1000.000000000000000 ) ;
#9526=VECTOR ( 'NONE', #10062, 1000.000000000000000 ) ;
#9528=EDGE_LOOP ( 'NONE', ( #58115, #10190, #40668, #65343, #31297, #32731 ) ) ;
#9586=EDGE_LOOP ( 'NONE', ( #6122, #39532 ) ) ;
#9599=CARTESIAN_POINT ( 'NONE',  ( 427.4999999999999432, 207.5000000000000284, 380.0000000000000000 ) ) ;
#9616=DIRECTION ( 'NONE',  ( -0.000000000000000000, 0.000000000000000000, -1.000000000000000000 ) ) ;
#9638=VERTEX_POINT ( 'NONE', #66433 ) ;
#9645=LINE ( 'NONE', #15263, #25245 ) ;
#9719=VERTEX_POINT ( 'NONE', #42437 ) ;
#9732=CARTESIAN_POINT ( 'NONE',  ( 209.3223706822284100, -1.426547569622074412E-15, 31.44247402469554942 ) ) ;
#9735=ORIENTED_EDGE ( 'NONE', *, *, #43488, .F. ) ;
#9748=VECTOR ( 'NONE', #47211, 1000.000000000000000 ) ;
#9757=DIRECTION ( 'NONE',  ( 0.000000000000000000, 0.000000000000000000, -1.000000000000000000 ) ) ;
#9788=DIRECTION ( 'NONE',  ( -0.000000000000000000, 0.000000000000000000, -1.000000000000000000 ) ) ;
#9794=DIRECTION ( 'NONE',  ( -1.000000000000000000, 0.000000000000000000, 0.000000000000000000 ) ) ;
#9864=FACE_OUTER_BOUND ( 'NONE', #28830, .T. ) ;
#9881=ORIENTED_EDGE ( 'NONE', *, *, #7578, .T. ) ;
#9912=VECTOR ( 'NONE', #23444, 1000.000000000000000 ) ;
#9935=EDGE_CURVE ( 'NONE', #1535, #22014, #40153, .T. ) ;
#9938=ADVANCED_FACE ( 'NONE', ( #23430 ), #29384, .F. ) ;
#9949=VERTEX_POINT ( 'NONE', #51195 ) ;
#9972=CARTESIAN_POINT ( 'NONE',  ( 144.4165763529819344, -26.99999999999998224, 138.9999999999999716 ) ) ;
#10007=ORIENTED_EDGE ( 'NONE', *, *, #56079, .F. ) ;
#10014=CARTESIAN_POINT ( 'NONE',  ( 0.000000000000000000, 0.000000000000000000, -2.000000000000000000 ) ) ;
#10045=ORIENTED_EDGE ( 'NONE', *, *, #23759, .T. ) ;
#10062=DIRECTION ( 'NONE',  ( 1.000000000000000000, -0.000000000000000000, 0.000000000000000000 ) ) ;
#10074=ADVANCED_FACE ( 'NONE', ( #46590 ), #52220, .F. ) ;
#10117=ORIENTED_EDGE ( 'NONE', *, *, #25425, .T. ) ;
#10132=ORIENTED_EDGE ( 'NONE', *, *, #35579, .T. ) ;
#10157=CARTESIAN_POINT ( 'NONE',  ( 422.4999999999999432, 207.5000000000000284, 0.000000000000000000 ) ) ;
#10185=DIRECTION ( 'NONE',  ( 0.000000000000000000, 0.000000000000000000, -1.000000000000000000 ) ) ;
#10190=ORIENTED_EDGE ( 'NONE', *, *, #8569, .T. ) ;
#10193=DIRECTION ( 'NONE',  ( 0.000000000000000000, 0.000000000000000000, -1.000000000000000000 ) ) ;
#10218=AXIS2_PLACEMENT_3D ( 'NONE', #33581, #66300, #34271 ) ;
#10227=CARTESIAN_POINT ( 'NONE',  ( 0.000000000000000000, 0.000000000000000000, 0.000000000000000000 ) ) ;
#10243=CARTESIAN_POINT ( 'NONE',  ( 109.9975424824652777, 296.0000000000000000, 418.0000000000000000 ) ) ;
#10288=DIRECTION ( 'NONE',  ( 1.000000000000000000, 0.000000000000000000, 0.000000000000000000 ) ) ;
#10293=DIRECTION ( 'NONE',  ( -0.000000000000000000, 1.000000000000000000, -0.000000000000000000 ) ) ;
#10300=VECTOR ( 'NONE', #67787, 1000.000000000000000 ) ;
#10327=CARTESIAN_POINT ( 'NONE',  ( 109.9975424824652634, 22.00669820036271673, 401.6295345748408181 ) ) ;
#10377=DIRECTION ( 'NONE',  ( -1.000000000000000000, 0.000000000000000000, 0.000000000000000000 ) ) ;
#10398=DIRECTION ( 'NONE',  ( -0.000000000000000000, -1.000000000000000000, 0.000000000000000000 ) ) ;
#10402=ORIENTED_EDGE ( 'NONE', *, *, #21208, .T. ) ;
#10415=ORIENTED_EDGE ( 'NONE', *, *, #48308, .T. ) ;
#10430=CARTESIAN_POINT ( 'NONE',  ( 141.9165763529819344, 242.0000000000000000, 108.9999999999999858 ) ) ;
#10461=VECTOR ( 'NONE', #23119, 1000.000000000000000 ) ;
#10473=VERTEX_POINT ( 'NONE', #19429 ) ;
#10486=ORIENTED_EDGE ( 'NONE', *, *, #11040, .F. ) ;
#10491=AXIS2_PLACEMENT_3D ( 'NONE', #7891, #24068, #2272 ) ;
#10503=FACE_OUTER_BOUND ( 'NONE', #21510, .T. ) ;
#10516=FACE_BOUND ( 'NONE', #1797, .T. ) ;
#10521=ORIENTED_EDGE ( 'NONE', *, *, #13717, .F. ) ;
#10552=FACE_OUTER_BOUND ( 'NONE', #4431, .T. ) ;
#10559=ORIENTED_EDGE ( 'NONE', *, *, #15348, .T. ) ;
#10570=DIRECTION ( 'NONE',  ( -0.000000000000000000, -0.000000000000000000, 1.000000000000000000 ) ) ;
#10589=CARTESIAN_POINT ( 'NONE',  ( 311.9975424824652350, 0.000000000000000000, 255.6641978984094408 ) ) ;
#10620=CARTESIAN_POINT ( 'NONE',  ( 444.9999999999999432, -35.00000000000000000, 378.0000000000000000 ) ) ;
#10625=LINE ( 'NONE', #64444, #31922 ) ;
#10629=PLANE ( 'NONE',  #40535 ) ;
#10636=EDGE_CURVE ( 'NONE', #24965, #59809, #27824, .T. ) ;
#10644=EDGE_CURVE ( 'NONE', #44856, #33368, #38374, .T. ) ;
#10652=CARTESIAN_POINT ( 'NONE',  ( 109.9975424824652634, 18.08738615523480675, 402.4289050101931480 ) ) ;
#10679=CARTESIAN_POINT ( 'NONE',  ( 188.9999999999999432, -57.00000000000007816, 72.99999999999998579 ) ) ;
#10689=DIRECTION ( 'NONE',  ( -1.000000000000000000, 0.000000000000000000, 0.000000000000000000 ) ) ;
#10711=ORIENTED_EDGE ( 'NONE', *, *, #31931, .F. ) ;
#10739=VECTOR ( 'NONE', #20213, 1000.000000000000000 ) ;
#10754=EDGE_LOOP ( 'NONE', ( #16020, #40102, #33403, #23452 ) ) ;
#10778=PLANE ( 'NONE',  #59853 ) ;
#10800=AXIS2_PLACEMENT_3D ( 'NONE', #4015, #20185, #57825 ) ;
#10803=CARTESIAN_POINT ( 'NONE',  ( 141.9165763529819344, 192.0000000000000000, 129.0000000000000284 ) ) ;
#10810=VECTOR ( 'NONE', #46773, 1000.000000000000000 ) ;
#10824=EDGE_CURVE ( 'NONE', #21633, #31241, #36827, .T. ) ;
#10841=CIRCLE ( 'NONE', #53516, 245.3095347406802489 ) ;
#10849=ORIENTED_EDGE ( 'NONE', *, *, #56442, .F. ) ;
#10854=EDGE_CURVE ( 'NONE', #9719, #21528, #61537, .T. ) ;
#10860=DIRECTION ( 'NONE',  ( 0.000000000000000000, 1.000000000000000000, 0.000000000000000000 ) ) ;
#10865=DIRECTION ( 'NONE',  ( -1.000000000000000000, 0.000000000000000000, -0.000000000000000000 ) ) ;
#10893=ORIENTED_EDGE ( 'NONE', *, *, #37724, .T. ) ;
#10906=PLANE ( 'NONE',  #62624 ) ;
#10924=AXIS2_PLACEMENT_3D ( 'NONE', #2453, #60494, #29187 ) ;
#10937=EDGE_LOOP ( 'NONE', ( #52914, #66851, #14980, #28136 ) ) ;
#10938=EDGE_CURVE ( 'NONE', #38117, #51614, #60367, .T. ) ;
#10958=CARTESIAN_POINT ( 'NONE',  ( 109.9975424824652634, 295.8720703627916464, 535.5371946177799600 ) ) ;
#10974=CYLINDRICAL_SURFACE ( 'NONE', #18393, 5.000000000000000888 ) ;
#10983=DIRECTION ( 'NONE',  ( -1.000000000000000000, 0.000000000000000000, 0.000000000000000000 ) ) ;
#10988=ORIENTED_EDGE ( 'NONE', *, *, #26678, .F. ) ;
#10996=AXIS2_PLACEMENT_3D ( 'NONE', #56114, #29383, #40621 ) ;
#11002=VECTOR ( 'NONE', #44534, 1000.000000000000000 ) ;
#11022=DIRECTION ( 'NONE',  ( 0.000000000000000000, 0.000000000000000000, -1.000000000000000000 ) ) ;
#11040=EDGE_CURVE ( 'NONE', #55571, #44856, #16581, .T. ) ;
#11067=CARTESIAN_POINT ( 'NONE',  ( -2.000000000000000000, -2.000000000000000000, 0.000000000000000000 ) ) ;
#11075=EDGE_LOOP ( 'NONE', ( #20004, #53474, #62375, #7123, #60136, #46985, #59718, #34816 ) ) ;
#11088=CARTESIAN_POINT ( 'NONE',  ( 141.9165763529819344, 242.0000000000000000, 129.0000000000000000 ) ) ;
#11103=EDGE_CURVE ( 'NONE', #43378, #57196, #55074, .T. ) ;
#11118=VERTEX_POINT ( 'NONE', #32249 ) ;
#11126=ADVANCED_FACE ( 'NONE', ( #50851 ), #18847, .T. ) ;
#11132=ORIENTED_EDGE ( 'NONE', *, *, #23759, .F. ) ;
#11136=CARTESIAN_POINT ( 'NONE',  ( 188.9999999999999432, 225.0000000000000000, 0.000000000000000000 ) ) ;
#11170=ORIENTED_EDGE ( 'NONE', *, *, #37793, .T. ) ;
#11171=CARTESIAN_POINT ( 'NONE',  ( 230.9999999999999432, 0.000000000000000000, -2.000000000000000000 ) ) ;
#11176=EDGE_CURVE ( 'NONE', #41448, #55844, #1986, .T. ) ;
#11194=ORIENTED_EDGE ( 'NONE', *, *, #17132, .T. ) ;
#11209=DIRECTION ( 'NONE',  ( 0.000000000000000000, 0.000000000000000000, -1.000000000000000000 ) ) ;
#11262=EDGE_CURVE ( 'NONE', #28403, #58183, #46959, .T. ) ;
#11319=ADVANCED_FACE ( 'NONE', ( #44084 ), #38475, .F. ) ;
#11332=EDGE_CURVE ( 'NONE', #16701, #21755, #63840, .T. ) ;
#11360=DIRECTION ( 'NONE',  ( 0.000000000000000000, -1.000000000000000000, 0.000000000000000000 ) ) ;
#11403=DIRECTION ( 'NONE',  ( -0.000000000000000000, -0.000000000000000000, -1.000000000000000000 ) ) ;
#11432=ORIENTED_EDGE ( 'NONE', *, *, #37152, .F. ) ;
#11447=DIRECTION ( 'NONE',  ( 0.000000000000000000, 0.000000000000000000, -1.000000000000000000 ) ) ;
#11462=LINE ( 'NONE', #32589, #28432 ) ;
#11501=CARTESIAN_POINT ( 'NONE',  ( 311.9975424824652350, 170.0000000000000284, 354.1673509436691347 ) ) ;
#11543=DIRECTION ( 'NONE',  ( -0.000000000000000000, -0.000000000000000000, -1.000000000000000000 ) ) ;
#11545=VECTOR ( 'NONE', #55450, 1000.000000000000000 ) ;
#11551=VECTOR ( 'NONE', #61003, 1000.000000000000000 ) ;
#11610=VERTEX_POINT ( 'NONE', #18686 ) ;
#11624=FACE_OUTER_BOUND ( 'NONE', #49379, .T. ) ;
#11641=VERTEX_POINT ( 'NONE', #39108 ) ;
#11642=EDGE_CURVE ( 'NONE', #68503, #49852, #2507, .T. ) ;
#11698=VERTEX_POINT ( 'NONE', #2166 ) ;
#11702=CARTESIAN_POINT ( 'NONE',  ( 412.0000000000000000, -2.000000000000000000, 380.0000000000000000 ) ) ;
#11710=VECTOR ( 'NONE', #26587, 1000.000000000000000 ) ;
#11711=DIRECTION ( 'NONE',  ( 0.000000000000000000, 0.000000000000000000, 1.000000000000000000 ) ) ;
#11713=DIRECTION ( 'NONE',  ( -1.000000000000000000, 0.000000000000000000, 0.000000000000000000 ) ) ;
#11728=FACE_OUTER_BOUND ( 'NONE', #41382, .T. ) ;
#11761=( GEOMETRIC_REPRESENTATION_CONTEXT ( 3 ) GLOBAL_UNCERTAINTY_ASSIGNED_CONTEXT ( ( #50093 ) ) GLOBAL_UNIT_ASSIGNED_CONTEXT ( ( #61431, #56148, #17464 ) ) REPRESENTATION_CONTEXT ( 'NONE', 'WORKASPACE' ) );
#11778=VERTEX_POINT ( 'NONE', #34178 ) ;
#11796=CARTESIAN_POINT ( 'NONE',  ( 111.9975424824652634, 170.0000000000000284, 354.1673509436691347 ) ) ;
#11809=EDGE_CURVE ( 'NONE', #57714, #8357, #35203, .T. ) ;
#11811=DIRECTION ( 'NONE',  ( 1.000000000000000000, 0.000000000000000000, -0.000000000000000000 ) ) ;
#11852=VECTOR ( 'NONE', #54905, 1000.000000000000000 ) ;
#11879=VERTEX_POINT ( 'NONE', #26034 ) ;
#11890=EDGE_CURVE ( 'NONE', #46362, #8192, #56659, .T. ) ;
#11908=FACE_OUTER_BOUND ( 'NONE', #66461, .T. ) ;
#11954=EDGE_LOOP ( 'NONE', ( #34367, #18717 ) ) ;
#11955=ORIENTED_EDGE ( 'NONE', *, *, #37368, .F. ) ;
#11978=DIRECTION ( 'NONE',  ( 0.000000000000000000, 0.000000000000000000, -1.000000000000000000 ) ) ;
#11985=CARTESIAN_POINT ( 'NONE',  ( 111.9975424824652634, 20.00000000000003197, 536.6193948016162949 ) ) ;
#12023=CARTESIAN_POINT ( 'NONE',  ( 311.9975424824652350, 307.8795515535290974, 6.994434899193393562 ) ) ;
#12068=AXIS2_PLACEMENT_3D ( 'NONE', #11985, #37667, #27812 ) ;
#12139=LINE ( 'NONE', #49745, #23570 ) ;
#12140=EDGE_CURVE ( 'NONE', #60658, #57264, #39705, .T. ) ;
#12143=VERTEX_POINT ( 'NONE', #65753 ) ;
#12147=DIRECTION ( 'NONE',  ( -1.000000000000000000, 0.000000000000000000, 0.000000000000000000 ) ) ;
#12228=LINE ( 'NONE', #39652, #2126 ) ;
#12304=LINE ( 'NONE', #39385, #5830 ) ;
#12308=ORIENTED_EDGE ( 'NONE', *, *, #33768, .T. ) ;
#12310=ORIENTED_EDGE ( 'NONE', *, *, #6159, .T. ) ;
#12357=ORIENTED_EDGE ( 'NONE', *, *, #58353, .F. ) ;
#12390=ORIENTED_EDGE ( 'NONE', *, *, #36064, .T. ) ;
#12412=EDGE_CURVE ( 'NONE', #65444, #12143, #56757, .T. ) ;
#12416=EDGE_CURVE ( 'NONE', #21755, #48801, #29673, .T. ) ;
#12471=EDGE_CURVE ( 'NONE', #61576, #59809, #44689, .T. ) ;
#12472=ADVANCED_FACE ( 'NONE', ( #33088 ), #1424, .F. ) ;
#12483=ORIENTED_EDGE ( 'NONE', *, *, #28078, .T. ) ;
#12534=VERTEX_POINT ( 'NONE', #21824 ) ;
#12562=CARTESIAN_POINT ( 'NONE',  ( 444.9999999999999432, -35.00000000000000000, -2.000000000000000000 ) ) ;
#12570=LINE ( 'NONE', #65338, #5522 ) ;
#12579=CIRCLE ( 'NONE', #9209, 5.000000000000000888 ) ;
#12607=LINE ( 'NONE', #39683, #31749 ) ;
#12609=DIRECTION ( 'NONE',  ( -1.000000000000000000, 0.000000000000000000, 0.000000000000000000 ) ) ;
#12619=ORIENTED_EDGE ( 'NONE', *, *, #24226, .T. ) ;
#12632=ORIENTED_EDGE ( 'NONE', *, *, #36373, .T. ) ;
#12635=ORIENTED_EDGE ( 'NONE', *, *, #51653, .T. ) ;
#12638=DIRECTION ( 'NONE',  ( 0.000000000000000000, -1.000000000000000000, -1.385458760688113094E-14 ) ) ;
#12677=ORIENTED_EDGE ( 'NONE', *, *, #69390, .T. ) ;
#12707=ADVANCED_FACE ( 'NONE', ( #5995 ), #29, .F. ) ;
#12708=ORIENTED_EDGE ( 'NONE', *, *, #10854, .T. ) ;
#12719=ORIENTED_EDGE ( 'NONE', *, *, #46763, .F. ) ;
#12807=ORIENTED_EDGE ( 'NONE', *, *, #56224, .T. ) ;
#12838=CARTESIAN_POINT ( 'NONE',  ( 230.9999999999999432, 0.000000000000000000, 0.000000000000000000 ) ) ;
#12839=VECTOR ( 'NONE', #64526, 1000.000000000000000 ) ;
#12858=EDGE_CURVE ( 'NONE', #31241, #21633, #44666, .T. ) ;
#12877=CARTESIAN_POINT ( 'NONE',  ( 230.9999999999999432, 192.0000000000000000, 0.000000000000000000 ) ) ;
#12897=PLANE ( 'NONE',  #33004 ) ;
#12912=LINE ( 'NONE', #5865, #11545 ) ;
#12935=VECTOR ( 'NONE', #50668, 1000.000000000000000 ) ;
#12938=VECTOR ( 'NONE', #34200, 1000.000000000000114 ) ;
#12942=CARTESIAN_POINT ( 'NONE',  ( 0.000000000000000000, 0.000000000000000000, -2.000000000000000000 ) ) ;
#12945=ORIENTED_EDGE ( 'NONE', *, *, #66738, .F. ) ;
#12947=EDGE_CURVE ( 'NONE', #34313, #35904, #63649, .T. ) ;
#12996=LINE ( 'NONE', #13338, #8367 ) ;
#13022=DIRECTION ( 'NONE',  ( 0.000000000000000000, -0.000000000000000000, 1.000000000000000000 ) ) ;
#13027=FACE_OUTER_BOUND ( 'NONE', #36972, .T. ) ;
#13050=VERTEX_POINT ( 'NONE', #66438 ) ;
#13076=DIRECTION ( 'NONE',  ( 0.000000000000000000, 1.000000000000000000, 0.000000000000000000 ) ) ;
#13089=DIRECTION ( 'NONE',  ( -0.000000000000000000, -0.000000000000000000, -1.000000000000000000 ) ) ;
#13145=VECTOR ( 'NONE', #34094, 1000.000000000000000 ) ;
#13148=ORIENTED_EDGE ( 'NONE', *, *, #60502, .F. ) ;
#13181=LINE ( 'NONE', #39904, #30762 ) ;
#13211=VERTEX_POINT ( 'NONE', #41067 ) ;
#13218=DIRECTION ( 'NONE',  ( 0.000000000000000000, 0.000000000000000000, -1.000000000000000000 ) ) ;
#13231=DIRECTION ( 'NONE',  ( 0.000000000000000000, 0.000000000000000000, 1.000000000000000000 ) ) ;
#13232=AXIS2_PLACEMENT_3D ( 'NONE', #22531, #21479, #16208 ) ;
#13286=CARTESIAN_POINT ( 'NONE',  ( 230.9999999999999432, -57.00000000000007816, -2.000000000000000000 ) ) ;
#13287=ORIENTED_EDGE ( 'NONE', *, *, #57997, .T. ) ;
#13296=DIRECTION ( 'NONE',  ( 0.000000000000000000, 1.000000000000000000, 0.000000000000000000 ) ) ;
#13314=CARTESIAN_POINT ( 'NONE',  ( 427.4999999999999432, 207.5000000000000284, -2.000000000000000000 ) ) ;
#13321=AXIS2_PLACEMENT_3D ( 'NONE', #51249, #10293, #37041 ) ;
#13326=LINE ( 'NONE', #56930, #16373 ) ;
#13338=CARTESIAN_POINT ( 'NONE',  ( 409.0783954480986608, -1.426547569622074412E-15, 174.7010307253933377 ) ) ;
#13371=VECTOR ( 'NONE', #34034, 1000.000000000000000 ) ;
#13376=EDGE_CURVE ( 'NONE', #66758, #44768, #16748, .T. ) ;
#13436=LINE ( 'NONE', #2879, #61970 ) ;
#13452=ORIENTED_EDGE ( 'NONE', *, *, #59581, .F. ) ;
#13454=DIRECTION ( 'NONE',  ( 0.000000000000000000, 0.000000000000000000, -1.000000000000000000 ) ) ;
#13466=CARTESIAN_POINT ( 'NONE',  ( 141.9165763529819344, 242.0000000000000000, 129.0000000000000000 ) ) ;
#13467=VERTEX_POINT ( 'NONE', #58438 ) ;
#13480=FACE_OUTER_BOUND ( 'NONE', #58726, .T. ) ;
#13501=CARTESIAN_POINT ( 'NONE',  ( 144.4165763529819344, 225.8585178651493663, 138.9999999999999716 ) ) ;
#13517=EDGE_CURVE ( 'NONE', #55258, #4522, #22205, .T. ) ;
#13537=ORIENTED_EDGE ( 'NONE', *, *, #18891, .F. ) ;
#13596=EDGE_CURVE ( 'NONE', #1198, #19781, #47131, .T. ) ;
#13597=ORIENTED_EDGE ( 'NONE', *, *, #54935, .T. ) ;
#13598=AXIS2_PLACEMENT_3D ( 'NONE', #21256, #26194, #15977 ) ;
#13629=ORIENTED_EDGE ( 'NONE', *, *, #33270, .F. ) ;
#13633=AXIS2_PLACEMENT_3D ( 'NONE', #54174, #738, #32406 ) ;
#13644=DIRECTION ( 'NONE',  ( 0.000000000000000000, 0.000000000000000000, 1.000000000000000000 ) ) ;
#13662=DIRECTION ( 'NONE',  ( 0.000000000000000000, 0.000000000000000000, 1.000000000000000000 ) ) ;
#13666=DIRECTION ( 'NONE',  ( 0.000000000000000000, 0.000000000000000000, -1.000000000000000000 ) ) ;
#13672=DIRECTION ( 'NONE',  ( 0.000000000000000000, -1.385458760688113094E-14, 1.000000000000000000 ) ) ;
#13686=ORIENTED_EDGE ( 'NONE', *, *, #15787, .F. ) ;
#13688=AXIS2_PLACEMENT_3D ( 'NONE', #49231, #1067, #65435 ) ;
#13717=EDGE_CURVE ( 'NONE', #17316, #18390, #43558, .T. ) ;
#13718=DIRECTION ( 'NONE',  ( 0.000000000000000000, 0.000000000000000000, -1.000000000000000000 ) ) ;
#13739=ADVANCED_FACE ( 'NONE', ( #15803, #10516, #11908 ), #49525, .T. ) ;
#13740=VERTEX_POINT ( 'NONE', #54452 ) ;
#13754=CARTESIAN_POINT ( 'NONE',  ( 444.9999999999999432, -35.00000000000000000, -2.000000000000000000 ) ) ;
#13755=CARTESIAN_POINT ( 'NONE',  ( 188.9999999999999432, 225.0000000000000000, 72.99999999999998579 ) ) ;
#13761=ADVANCED_FACE ( 'NONE', ( #54811 ), #65386, .F. ) ;
#13766=PLANE ( 'NONE',  #15016 ) ;
#13843=VERTEX_POINT ( 'NONE', #16143 ) ;
#13844=CARTESIAN_POINT ( 'NONE',  ( 209.3223706822284100, 0.000000000000000000, 31.44247402469554942 ) ) ;
#13856=CARTESIAN_POINT ( 'NONE',  ( 209.3223706822284100, 18.00000000000002842, 31.44247402469554942 ) ) ;
#13863=DIRECTION ( 'NONE',  ( 0.000000000000000000, 0.000000000000000000, -1.000000000000000000 ) ) ;
#13982=VECTOR ( 'NONE', #42213, 1000.000000000000000 ) ;
#13983=VECTOR ( 'NONE', #1379, 1000.000000000000000 ) ;
#13994=DIRECTION ( 'NONE',  ( 0.000000000000000000, 1.000000000000000000, -0.000000000000000000 ) ) ;
#14033=CIRCLE ( 'NONE', #38729, 5.000000000000004441 ) ;
#14058=CARTESIAN_POINT ( 'NONE',  ( -35.00000000000002842, -35.00000000000000000, 380.0000000000000000 ) ) ;
#14063=FACE_OUTER_BOUND ( 'NONE', #36751, .T. ) ;
#14093=DIRECTION ( 'NONE',  ( 0.000000000000000000, 0.000000000000000000, -1.000000000000000000 ) ) ;
#14121=FACE_OUTER_BOUND ( 'NONE', #15384, .T. ) ;
#14125=DIRECTION ( 'NONE',  ( 1.000000000000000000, 0.000000000000000000, 0.000000000000000000 ) ) ;
#14130=VERTEX_POINT ( 'NONE', #42785 ) ;
#14131=FACE_BOUND ( 'NONE', #22026, .T. ) ;
#14137=FACE_BOUND ( 'NONE', #11954, .T. ) ;
#14171=ORIENTED_EDGE ( 'NONE', *, *, #11040, .T. ) ;
#14177=DIRECTION ( 'NONE',  ( 0.000000000000000000, -0.1086713087885527035, -0.9940777367219240102 ) ) ;
#14188=FACE_OUTER_BOUND ( 'NONE', #36364, .T. ) ;
#14212=DIRECTION ( 'NONE',  ( 0.000000000000000000, 1.000000000000000000, 0.000000000000000000 ) ) ;
#14271=PRODUCT_DEFINITION_SHAPE ( 'NONE', 'NONE',  #3950 ) ;
#14326=APPLICATION_CONTEXT ( 'automotive_design' ) ;
#14335=VECTOR ( 'NONE', #58347, 1000.000000000000000 ) ;
#14338=VECTOR ( 'NONE', #31714, 1000.000000000000000 ) ;
#14375=VERTEX_POINT ( 'NONE', #52238 ) ;
#14382=EDGE_CURVE ( 'NONE', #55222, #42236, #31474, .T. ) ;
#14398=DIRECTION ( 'NONE',  ( -1.000000000000000000, 0.000000000000000000, 0.000000000000000000 ) ) ;
#14446=DIRECTION ( 'NONE',  ( 0.000000000000000000, 0.000000000000000000, -1.000000000000000000 ) ) ;
#14536=EDGE_CURVE ( 'NONE', #11118, #69500, #38126, .T. ) ;
#14537=CIRCLE ( 'NONE', #4445, 5.000000000000004441 ) ;
#14554=EDGE_CURVE ( 'NONE', #41180, #40156, #33216, .T. ) ;
#14570=FACE_OUTER_BOUND ( 'NONE', #65985, .T. ) ;
#14597=ORIENTED_EDGE ( 'NONE', *, *, #67351, .F. ) ;
#14633=CIRCLE ( 'NONE', #4540, 5.000000000000004441 ) ;
#14640=VERTEX_POINT ( 'NONE', #29322 ) ;
#14650=LINE ( 'NONE', #26928, #11710 ) ;
#14700=CIRCLE ( 'NONE', #38239, 5.000000000000004441 ) ;
#14710=LINE ( 'NONE', #67846, #24282 ) ;
#14720=VERTEX_POINT ( 'NONE', #40915 ) ;
#14723=EDGE_CURVE ( 'NONE', #35609, #27646, #37092, .T. ) ;
#14736=AXIS2_PLACEMENT_3D ( 'NONE', #51853, #19493, #68048 ) ;
#14743=FACE_BOUND ( 'NONE', #26083, .T. ) ;
#14754=VERTEX_POINT ( 'NONE', #19811 ) ;
#14919=ORIENTED_EDGE ( 'NONE', *, *, #45838, .T. ) ;
#14939=CARTESIAN_POINT ( 'NONE',  ( -17.50000000000002842, -18.06806526123148160, 380.0000000000000000 ) ) ;
#14950=VERTEX_POINT ( 'NONE', #17906 ) ;
#14979=EDGE_CURVE ( 'NONE', #5170, #3478, #14700, .T. ) ;
#14980=ORIENTED_EDGE ( 'NONE', *, *, #48905, .T. ) ;
#14991=DIRECTION ( 'NONE',  ( -0.000000000000000000, -0.000000000000000000, 1.000000000000000000 ) ) ;
#15016=AXIS2_PLACEMENT_3D ( 'NONE', #40496, #66561, #61266 ) ;
#15052=CIRCLE ( 'NONE', #42009, 245.3095347406802773 ) ;
#15079=CARTESIAN_POINT ( 'NONE',  ( 141.9165763529819344, -52.00000000000000711, 129.0000000000000000 ) ) ;
#15091=ORIENTED_EDGE ( 'NONE', *, *, #10824, .F. ) ;
#15097=EDGE_CURVE ( 'NONE', #18335, #62679, #43853, .T. ) ;
#15100=DIRECTION ( 'NONE',  ( 0.000000000000000000, -0.000000000000000000, 1.000000000000000000 ) ) ;
#15113=ORIENTED_EDGE ( 'NONE', *, *, #14723, .F. ) ;
#15139=VECTOR ( 'NONE', #24152, 1000.000000000000000 ) ;
#15171=VERTEX_POINT ( 'NONE', #69533 ) ;
#15207=DIRECTION ( 'NONE',  ( -0.000000000000000000, -0.000000000000000000, -1.000000000000000000 ) ) ;
#15240=EDGE_CURVE ( 'NONE', #12534, #25214, #38225, .T. ) ;
#15263=CARTESIAN_POINT ( 'NONE',  ( 230.9999999999999432, 190.0000000000000000, 380.0000000000000000 ) ) ;
#15265=CARTESIAN_POINT ( 'NONE',  ( -17.50000000000002842, 207.5000000000000284, -2.000000000000000000 ) ) ;
#15270=( NAMED_UNIT ( * ) SI_UNIT ( $, .STERADIAN. ) SOLID_ANGLE_UNIT ( ) );
#15280=VECTOR ( 'NONE', #39291, 1000.000000000000000 ) ;
#15301=EDGE_CURVE ( 'NONE', #454, #2243, #40314, .T. ) ;
#15345=CARTESIAN_POINT ( 'NONE',  ( 427.4999999999999432, -18.06806526123148160, 378.0000000000000000 ) ) ;
#15347=DIRECTION ( 'NONE',  ( -1.000000000000000000, -0.000000000000000000, -0.000000000000000000 ) ) ;
#15348=EDGE_CURVE ( 'NONE', #57527, #13467, #45240, .T. ) ;
#15374=DIRECTION ( 'NONE',  ( -0.000000000000000000, -1.000000000000000000, -0.000000000000000000 ) ) ;
#15384=EDGE_LOOP ( 'NONE', ( #22541, #26204, #62690, #34851 ) ) ;
#15388=DIRECTION ( 'NONE',  ( 0.000000000000000000, 1.000000000000000000, 0.000000000000000000 ) ) ;
#15413=EDGE_CURVE ( 'NONE', #56653, #35195, #19550, .T. ) ;
#15416=CARTESIAN_POINT ( 'NONE',  ( 309.8720357909272707, 18.00000000000002842, 256.6193948016162381 ) ) ;
#15460=CARTESIAN_POINT ( 'NONE',  ( 259.4165763529819060, -27.00000000000000355, 128.9999999999999716 ) ) ;
#15465=LINE ( 'NONE', #43204, #5219 ) ;
#15474=DIRECTION ( 'NONE',  ( 1.000000000000000000, 0.000000000000000000, 0.000000000000000000 ) ) ;
#15482=( GEOMETRIC_REPRESENTATION_CONTEXT ( 3 ) GLOBAL_UNCERTAINTY_ASSIGNED_CONTEXT ( ( #44465 ) ) GLOBAL_UNIT_ASSIGNED_CONTEXT ( ( #3673, #46579, #15270 ) ) REPRESENTATION_CONTEXT ( 'NONE', 'WORKASPACE' ) );
#15488=EDGE_LOOP ( 'NONE', ( #19512, #10711, #1129, #53974 ) ) ;
#15492=DIRECTION ( 'NONE',  ( 0.000000000000000000, 1.000000000000000000, 0.000000000000000000 ) ) ;
#15558=LINE ( 'NONE', #10958, #32899 ) ;
#15566=DIRECTION ( 'NONE',  ( 1.000000000000000000, 0.000000000000000000, 0.000000000000000000 ) ) ;
#15571=VECTOR ( 'NONE', #64812, 1000.000000000000000 ) ;
#15577=ADVANCED_FACE ( 'NONE', ( #1923 ), #45153, .F. ) ;
#15591=DIRECTION ( 'NONE',  ( -1.000000000000000000, 0.000000000000000000, -0.000000000000000000 ) ) ;
#15600=DIRECTION ( 'NONE',  ( 1.000000000000000000, 0.000000000000000000, 0.000000000000000000 ) ) ;
#15736=CARTESIAN_POINT ( 'NONE',  ( -35.00000000000002842, 225.0000000000000000, -2.000000000000000000 ) ) ;
#15740=CARTESIAN_POINT ( 'NONE',  ( 444.9999999999999432, -35.00000000000000000, 0.000000000000000000 ) ) ;
#15747=CARTESIAN_POINT ( 'NONE',  ( 230.9999999999999432, -35.00000000000000000, -2.000000000000000000 ) ) ;
#15750=ORIENTED_EDGE ( 'NONE', *, *, #13596, .T. ) ;
#15753=LINE ( 'NONE', #37900, #22818 ) ;
#15787=EDGE_CURVE ( 'NONE', #39050, #16169, #60783, .T. ) ;
#15795=ORIENTED_EDGE ( 'NONE', *, *, #63925, .T. ) ;
#15803=FACE_BOUND ( 'NONE', #45179, .T. ) ;
#15808=EDGE_LOOP ( 'NONE', ( #11170, #41906 ) ) ;
#15834=ORIENTED_EDGE ( 'NONE', *, *, #34487, .F. ) ;
#15885=AXIS2_PLACEMENT_3D ( 'NONE', #59987, #23074, #11447 ) ;
#15920=DIRECTION ( 'NONE',  ( 1.000000000000000000, 0.000000000000000000, 0.000000000000000000 ) ) ;
#15956=EDGE_CURVE ( 'NONE', #5435, #20075, #51966, .T. ) ;
#15977=DIRECTION ( 'NONE',  ( 0.000000000000000000, -0.000000000000000000, 1.000000000000000000 ) ) ;
#15986=EDGE_LOOP ( 'NONE', ( #61363, #31722, #68845, #43596 ) ) ;
#15992=ORIENTED_EDGE ( 'NONE', *, *, #20705, .T. ) ;
#16020=ORIENTED_EDGE ( 'NONE', *, *, #33633, .F. ) ;
#16021=DIRECTION ( 'NONE',  ( 0.000000000000000000, -1.000000000000000000, 0.000000000000000000 ) ) ;
#16054=ORIENTED_EDGE ( 'NONE', *, *, #30902, .F. ) ;
#16081=CARTESIAN_POINT ( 'NONE',  ( 266.9165763529819628, -52.00000000000000711, 128.9999999999999716 ) ) ;
#16098=ORIENTED_EDGE ( 'NONE', *, *, #13517, .T. ) ;
#16121=DIRECTION ( 'NONE',  ( 0.000000000000000000, 1.000000000000000000, 0.000000000000000000 ) ) ;
#16122=VERTEX_POINT ( 'NONE', #61057 ) ;
#16143=CARTESIAN_POINT ( 'NONE',  ( 111.9975424824653487, 172.0000000000000284, 256.6193948016162381 ) ) ;
#16169=VERTEX_POINT ( 'NONE', #18846 ) ;
#16176=VECTOR ( 'NONE', #20764, 1000.000000000000000 ) ;
#16208=DIRECTION ( 'NONE',  ( -1.000000000000000000, 0.000000000000000000, 0.000000000000000000 ) ) ;
#16234=VECTOR ( 'NONE', #15347, 1000.000000000000000 ) ;
#16267=ADVANCED_FACE ( 'NONE', ( #52577 ), #4729, .T. ) ;
#16306=ORIENTED_EDGE ( 'NONE', *, *, #66591, .F. ) ;
#16359=EDGE_CURVE ( 'NONE', #3478, #5170, #59665, .T. ) ;
#16372=DIRECTION ( 'NONE',  ( -0.000000000000000000, -1.000000000000000000, -0.000000000000000000 ) ) ;
#16373=VECTOR ( 'NONE', #50952, 1000.000000000000000 ) ;
#16375=LINE ( 'NONE', #59274, #44301 ) ;
#16385=ORIENTED_EDGE ( 'NONE', *, *, #52861, .T. ) ;
#16417=ORIENTED_EDGE ( 'NONE', *, *, #39722, .T. ) ;
#16459=CARTESIAN_POINT ( 'NONE',  ( 0.000000000000000000, 296.0000000000000000, 0.000000000000000000 ) ) ;
#16465=CARTESIAN_POINT ( 'NONE',  ( 444.9999999999999432, 225.0000000000000000, -2.000000000000000000 ) ) ;
#16467=AXIS2_PLACEMENT_3D ( 'NONE', #49523, #7688, #49170 ) ;
#16482=VERTEX_POINT ( 'NONE', #42628 ) ;
#16528=CARTESIAN_POINT ( 'NONE',  ( 209.9999999999999716, 192.0000000000000000, 93.99999999999998579 ) ) ;
#16536=DIRECTION ( 'NONE',  ( 1.000000000000000000, 0.000000000000000000, -0.000000000000000000 ) ) ;
#16539=CARTESIAN_POINT ( 'NONE',  ( 109.9975424824652634, 295.6904194069557548, 539.5330678552892323 ) ) ;
#16581=CIRCLE ( 'NONE', #40194, 245.3095347406802773 ) ;
#16583=ORIENTED_EDGE ( 'NONE', *, *, #17292, .F. ) ;
#16606=DIRECTION ( 'NONE',  ( 0.000000000000000000, -0.02271222823333339177, 0.9997420440737084801 ) ) ;
#16627=CARTESIAN_POINT ( 'NONE',  ( 111.9975424824652634, 20.00000000000003197, 256.6193948016162381 ) ) ;
#16634=LINE ( 'NONE', #19587, #32866 ) ;
#16640=DIRECTION ( 'NONE',  ( 1.000000000000000000, 0.000000000000000000, 0.000000000000000000 ) ) ;
#16643=PLANE ( 'NONE',  #33831 ) ;
#16695=ORIENTED_EDGE ( 'NONE', *, *, #59785, .T. ) ;
#16701=VERTEX_POINT ( 'NONE', #20748 ) ;
#16706=ORIENTED_EDGE ( 'NONE', *, *, #44302, .F. ) ;
#16728=ORIENTED_EDGE ( 'NONE', *, *, #66713, .F. ) ;
#16748=CIRCLE ( 'NONE', #4410, 246.3582898394607241 ) ;
#16750=DIRECTION ( 'NONE',  ( 0.000000000000000000, 0.000000000000000000, -1.000000000000000000 ) ) ;
#16829=DIRECTION ( 'NONE',  ( -1.000000000000000000, 0.000000000000000000, 0.000000000000000000 ) ) ;
#16865=DIRECTION ( 'NONE',  ( 0.000000000000000000, 0.000000000000000000, -1.000000000000000000 ) ) ;
#16879=PLANE ( 'NONE',  #64442 ) ;
#16882=ADVANCED_FACE ( 'NONE', ( #17902 ), #66456, .T. ) ;
#16922=CARTESIAN_POINT ( 'NONE',  ( 0.000000000000000000, 0.000000000000000000, 380.0000000000000000 ) ) ;
#16981=DIRECTION ( 'NONE',  ( -1.000000000000000000, 0.000000000000000000, 2.775557561562891844E-16 ) ) ;
#16984=FACE_OUTER_BOUND ( 'NONE', #6561, .T. ) ;
#17016=AXIS2_PLACEMENT_3D ( 'NONE', #1854, #44753, #34562 ) ;
#17047=LINE ( 'NONE', #60325, #19563 ) ;
#17054=DIRECTION ( 'NONE',  ( -1.000000000000000000, 0.000000000000000000, 0.000000000000000000 ) ) ;
#17064=ORIENTED_EDGE ( 'NONE', *, *, #23131, .F. ) ;
#17088=DIRECTION ( 'NONE',  ( -1.000000000000000000, 0.000000000000000000, 0.000000000000000000 ) ) ;
#17096=CARTESIAN_POINT ( 'NONE',  ( 409.0783954480987745, 190.0000000000000000, 174.7010307253933092 ) ) ;
#17097=DIRECTION ( 'NONE',  ( -0.000000000000000000, -1.000000000000000000, 0.000000000000000000 ) ) ;
#17111=LINE ( 'NONE', #60029, #37916 ) ;
#17118=DIRECTION ( 'NONE',  ( -0.000000000000000000, -1.000000000000000000, -0.000000000000000000 ) ) ;
#17132=EDGE_CURVE ( 'NONE', #68787, #51614, #36159, .T. ) ;
#17141=PLANE ( 'NONE',  #40700 ) ;
#17147=ORIENTED_EDGE ( 'NONE', *, *, #54778, .F. ) ;
#17164=EDGE_LOOP ( 'NONE', ( #5083, #6954, #53341, #53385 ) ) ;
#17165=ORIENTED_EDGE ( 'NONE', *, *, #45838, .F. ) ;
#17167=DIRECTION ( 'NONE',  ( 0.000000000000000000, 0.000000000000000000, -1.000000000000000000 ) ) ;
#17169=DIRECTION ( 'NONE',  ( -0.000000000000000000, -0.000000000000000000, -1.000000000000000000 ) ) ;
#17201=EDGE_CURVE ( 'NONE', #30930, #9949, #51985, .T. ) ;
#17205=EDGE_LOOP ( 'NONE', ( #19991, #26235, #26728, #57821, #46100, #14171, #53172, #19, #60739, #40724, #18457, #14597 ) ) ;
#17235=CIRCLE ( 'NONE', #34136, 5.000000000000004441 ) ;
#17288=CARTESIAN_POINT ( 'NONE',  ( 427.4999999999999432, 207.5000000000000284, 378.0000000000000000 ) ) ;
#17292=EDGE_CURVE ( 'NONE', #39465, #8984, #43745, .T. ) ;
#17302=CYLINDRICAL_SURFACE ( 'NONE', #47535, 5.000000000000000888 ) ;
#17308=ORIENTED_EDGE ( 'NONE', *, *, #27041, .T. ) ;
#17316=VERTEX_POINT ( 'NONE', #50088 ) ;
#17336=CARTESIAN_POINT ( 'NONE',  ( 209.9999999999999716, 192.0000000000000000, 72.99999999999998579 ) ) ;
#17339=CARTESIAN_POINT ( 'NONE',  ( 311.9975424824652350, 20.00000000000003197, 536.6193948016162949 ) ) ;
#17402=ORIENTED_EDGE ( 'NONE', *, *, #67514, .T. ) ;
#17454=DIRECTION ( 'NONE',  ( -0.000000000000000000, 1.000000000000000000, 0.000000000000000000 ) ) ;
#17456=CARTESIAN_POINT ( 'NONE',  ( 0.000000000000000000, 190.0000000000000000, 161.3522585083728700 ) ) ;
#17464=( NAMED_UNIT ( * ) SI_UNIT ( $, .STERADIAN. ) SOLID_ANGLE_UNIT ( ) );
#17486=CARTESIAN_POINT ( 'NONE',  ( 313.9975424824652350, 295.8720703627916464, 535.5371946177799600 ) ) ;
#17500=CARTESIAN_POINT ( 'NONE',  ( 266.9165763529819628, -52.00000000000000711, 128.9999999999999716 ) ) ;
#17501=ORIENTED_EDGE ( 'NONE', *, *, #46286, .T. ) ;
#17535=LINE ( 'NONE', #23175, #36340 ) ;
#17622=LINE ( 'NONE', #61233, #5173 ) ;
#17669=ORIENTED_EDGE ( 'NONE', *, *, #7254, .F. ) ;
#17710=ORIENTED_EDGE ( 'NONE', *, *, #9935, .F. ) ;
#17757=AXIS2_PLACEMENT_3D ( 'NONE', #6812, #53597, #6108 ) ;
#17806=ORIENTED_EDGE ( 'NONE', *, *, #5955, .T. ) ;
#17812=CYLINDRICAL_SURFACE ( 'NONE', #40787, 245.3095347406802205 ) ;
#17835=CARTESIAN_POINT ( 'NONE',  ( 209.9999999999999716, -57.00000000000007816, 93.99999999999998579 ) ) ;
#17883=EDGE_LOOP ( 'NONE', ( #37970, #45888, #31388, #36630 ) ) ;
#17902=FACE_OUTER_BOUND ( 'NONE', #68575, .T. ) ;
#17906=CARTESIAN_POINT ( 'NONE',  ( 311.9975424824652350, 20.00000000000003197, 256.6193948016162381 ) ) ;
#17924=ORIENTED_EDGE ( 'NONE', *, *, #64817, .F. ) ;
#17959=CARTESIAN_POINT ( 'NONE',  ( 311.9975424824652350, 170.0000000000000284, 536.6193948016162949 ) ) ;
#17967=VERTEX_POINT ( 'NONE', #2614 ) ;
#18015=VERTEX_POINT ( 'NONE', #27780 ) ;
#18017=CARTESIAN_POINT ( 'NONE',  ( 311.9975424824652350, 296.0000000000000000, 420.0000000000000000 ) ) ;
#18090=ORIENTED_EDGE ( 'NONE', *, *, #43488, .T. ) ;
#18097=CARTESIAN_POINT ( 'NONE',  ( 230.9999999999999432, 225.0000000000000000, -2.000000000000000000 ) ) ;
#18108=ORIENTED_EDGE ( 'NONE', *, *, #38584, .F. ) ;
#18122=EDGE_CURVE ( 'NONE', #31482, #13050, #12304, .T. ) ;
#18142=ADVANCED_FACE ( 'NONE', ( #55555 ), #50626, .F. ) ;
#18143=CARTESIAN_POINT ( 'NONE',  ( 311.9975424824652350, 307.8795515535290974, 6.994434899193393562 ) ) ;
#18167=PLANE ( 'NONE',  #46464 ) ;
#18177=CARTESIAN_POINT ( 'NONE',  ( 230.9999999999999432, 190.0000000000000000, 72.99999999999998579 ) ) ;
#18208=DIRECTION ( 'NONE',  ( 0.000000000000000000, 0.000000000000000000, -1.000000000000000000 ) ) ;
#18215=VECTOR ( 'NONE', #67203, 1000.000000000000000 ) ;
#18254=ORIENTED_EDGE ( 'NONE', *, *, #37790, .T. ) ;
#18266=EDGE_LOOP ( 'NONE', ( #12719, #17064, #44879, #58736 ) ) ;
#18270=VECTOR ( 'NONE', #27351, 1000.000000000000000 ) ;
#18332=CYLINDRICAL_SURFACE ( 'NONE', #29699, 5.000000000000004441 ) ;
#18335=VERTEX_POINT ( 'NONE', #25303 ) ;
#18381=ORIENTED_EDGE ( 'NONE', *, *, #56224, .F. ) ;
#18389=EDGE_LOOP ( 'NONE', ( #26028, #25915, #68270, #1705, #65220, #49982 ) ) ;
#18390=VERTEX_POINT ( 'NONE', #41812 ) ;
#18393=AXIS2_PLACEMENT_3D ( 'NONE', #64098, #53179, #58465 ) ;
#18444=EDGE_CURVE ( 'NONE', #454, #40730, #65339, .T. ) ;
#18457=ORIENTED_EDGE ( 'NONE', *, *, #68283, .T. ) ;
#18464=DIRECTION ( 'NONE',  ( 1.000000000000000000, 0.000000000000000000, 0.000000000000000000 ) ) ;
#18466=CARTESIAN_POINT ( 'NONE',  ( 422.4999999999999432, -18.06806526123148160, 378.0000000000000000 ) ) ;
#18473=LINE ( 'NONE', #39921, #64588 ) ;
#18498=CARTESIAN_POINT ( 'NONE',  ( 209.3223706822284100, 0.000000000000000000, 31.44247402469554942 ) ) ;
#18535=EDGE_CURVE ( 'NONE', #34756, #48801, #39441, .T. ) ;
#18552=EDGE_LOOP ( 'NONE', ( #65546, #9077, #16706, #1228 ) ) ;
#18579=CARTESIAN_POINT ( 'NONE',  ( 111.9975424824652634, 295.8720703627916464, 535.5371946177799600 ) ) ;
#18623=EDGE_CURVE ( 'NONE', #61739, #5291, #28183, .T. ) ;
#18636=CARTESIAN_POINT ( 'NONE',  ( 109.9975424824652634, 172.0000000000001705, 529.9060149868646477 ) ) ;
#18638=VECTOR ( 'NONE', #62079, 1000.000000000000000 ) ;
#18651=EDGE_LOOP ( 'NONE', ( #3213, #53932, #7657, #61442 ) ) ;
#18654=CIRCLE ( 'NONE', #57969, 245.3095347406802773 ) ;
#18686=CARTESIAN_POINT ( 'NONE',  ( 141.9165763529819344, 242.0000000000000000, 129.0000000000000000 ) ) ;
#18696=CIRCLE ( 'NONE', #62477, 5.000000000000004441 ) ;
#18717=ORIENTED_EDGE ( 'NONE', *, *, #10824, .T. ) ;
#18727=ORIENTED_EDGE ( 'NONE', *, *, #27059, .T. ) ;
#18758=ORIENTED_EDGE ( 'NONE', *, *, #8619, .T. ) ;
#18764=CARTESIAN_POINT ( 'NONE',  ( 264.4165763529819628, -27.00000000000000355, 128.9999999999999716 ) ) ;
#18795=CARTESIAN_POINT ( 'NONE',  ( 427.4999999999999432, -18.06806526123148160, 0.000000000000000000 ) ) ;
#18796=LINE ( 'NONE', #12838, #63686 ) ;
#18797=AXIS2_PLACEMENT_3D ( 'NONE', #53563, #37742, #55572 ) ;
#18805=AXIS2_PLACEMENT_3D ( 'NONE', #68072, #67721, #25509 ) ;
#18829=ORIENTED_EDGE ( 'NONE', *, *, #11809, .F. ) ;
#18846=CARTESIAN_POINT ( 'NONE',  ( 422.4999999999999432, -18.06806526123148160, -2.000000000000000000 ) ) ;
#18847=PLANE ( 'NONE',  #59301 ) ;
#18855=CARTESIAN_POINT ( 'NONE',  ( -17.50000000000002842, -18.06806526123148160, 0.000000000000000000 ) ) ;
#18878=VERTEX_POINT ( 'NONE', #30393 ) ;
#18884=ORIENTED_EDGE ( 'NONE', *, *, #19290, .T. ) ;
#18891=EDGE_CURVE ( 'NONE', #65005, #66949, #21455, .T. ) ;
#18897=FACE_BOUND ( 'NONE', #66177, .T. ) ;
#18931=EDGE_CURVE ( 'NONE', #7345, #53458, #37382, .T. ) ;
#18955=CARTESIAN_POINT ( 'NONE',  ( 109.9975424824652634, 22.00669820036271673, 401.6295345748408181 ) ) ;
#18979=PLANE ( 'NONE',  #68949 ) ;
#19046=ADVANCED_FACE ( 'NONE', ( #32462 ), #6060, .T. ) ;
#19084=ORIENTED_EDGE ( 'NONE', *, *, #48395, .T. ) ;
#19097=ORIENTED_EDGE ( 'NONE', *, *, #12140, .T. ) ;
#19109=ORIENTED_EDGE ( 'NONE', *, *, #16359, .F. ) ;
#19143=ORIENTED_EDGE ( 'NONE', *, *, #15097, .T. ) ;
#19147=DIRECTION ( 'NONE',  ( 1.000000000000000000, 0.000000000000000000, 0.000000000000000000 ) ) ;
#19154=LINE ( 'NONE', #40608, #37651 ) ;
#19168=FACE_OUTER_BOUND ( 'NONE', #27680, .T. ) ;
#19207=AXIS2_PLACEMENT_3D ( 'NONE', #24232, #44973, #13662 ) ;
#19212=ADVANCED_FACE ( 'NONE', ( #63360 ), #68628, .F. ) ;
#19278=DIRECTION ( 'NONE',  ( -0.000000000000000000, -0.000000000000000000, -1.000000000000000000 ) ) ;
#19290=EDGE_CURVE ( 'NONE', #18878, #11641, #64182, .T. ) ;
#19297=ORIENTED_EDGE ( 'NONE', *, *, #23049, .F. ) ;
#19313=AXIS2_PLACEMENT_3D ( 'NONE', #24971, #55936, #7754 ) ;
#19343=DIRECTION ( 'NONE',  ( -0.000000000000000000, -0.000000000000000000, 1.000000000000000000 ) ) ;
#19344=ORIENTED_EDGE ( 'NONE', *, *, #56470, .F. ) ;
#19360=EDGE_CURVE ( 'NONE', #32729, #18015, #63193, .T. ) ;
#19383=ORIENTED_EDGE ( 'NONE', *, *, #67534, .F. ) ;
#19429=CARTESIAN_POINT ( 'NONE',  ( 230.9999999999999432, -35.00000000000000000, -2.000000000000000000 ) ) ;
#19467=FACE_OUTER_BOUND ( 'NONE', #24063, .T. ) ;
#19493=DIRECTION ( 'NONE',  ( -0.000000000000000000, -0.000000000000000000, 1.000000000000000000 ) ) ;
#19494=DIRECTION ( 'NONE',  ( 1.000000000000000000, 0.000000000000000000, 0.000000000000000000 ) ) ;
#19512=ORIENTED_EDGE ( 'NONE', *, *, #10938, .F. ) ;
#19514=ORIENTED_EDGE ( 'NONE', *, *, #11890, .T. ) ;
#19535=DIRECTION ( 'NONE',  ( -0.000000000000000000, -0.000000000000000000, -1.000000000000000000 ) ) ;
#19550=LINE ( 'NONE', #26209, #36046 ) ;
#19563=VECTOR ( 'NONE', #18464, 1000.000000000000000 ) ;
#19568=CARTESIAN_POINT ( 'NONE',  ( 259.4165763529819060, 225.8585178651493948, 108.9999999999999858 ) ) ;
#19587=CARTESIAN_POINT ( 'NONE',  ( 313.9975424824652350, 18.00000000000002842, 536.6193948016162949 ) ) ;
#19647=ORIENTED_EDGE ( 'NONE', *, *, #20870, .T. ) ;
#19653=VECTOR ( 'NONE', #45564, 1000.000000000000000 ) ;
#19744=CIRCLE ( 'NONE', #52282, 5.000000000000000888 ) ;
#19756=ORIENTED_EDGE ( 'NONE', *, *, #33768, .F. ) ;
#19758=ORIENTED_EDGE ( 'NONE', *, *, #32916, .F. ) ;
#19764=ORIENTED_EDGE ( 'NONE', *, *, #11332, .T. ) ;
#19781=VERTEX_POINT ( 'NONE', #5728 ) ;
#19797=DIRECTION ( 'NONE',  ( -1.000000000000000000, 0.000000000000000000, 0.000000000000000000 ) ) ;
#19798=ORIENTED_EDGE ( 'NONE', *, *, #25580, .T. ) ;
#19806=ADVANCED_FACE ( 'NONE', ( #43702 ), #33536, .F. ) ;
#19811=CARTESIAN_POINT ( 'NONE',  ( 111.9975424824652634, 170.0000000000000284, 354.1673509436691347 ) ) ;
#19837=DIRECTION ( 'NONE',  ( 1.000000000000000000, 0.000000000000000000, 0.000000000000000000 ) ) ;
#19847=CARTESIAN_POINT ( 'NONE',  ( 309.8720357909272707, 18.00000000000002842, 256.6193948016162381 ) ) ;
#19848=PLANE ( 'NONE',  #56098 ) ;
#19864=EDGE_CURVE ( 'NONE', #8603, #51213, #40686, .T. ) ;
#19873=ORIENTED_EDGE ( 'NONE', *, *, #33614, .T. ) ;
#19884=DIRECTION ( 'NONE',  ( -1.000000000000000000, 0.000000000000000000, 0.000000000000000000 ) ) ;
#19897=CIRCLE ( 'NONE', #53556, 164.5210298272983778 ) ;
#19909=ORIENTED_EDGE ( 'NONE', *, *, #32481, .F. ) ;
#19914=FACE_OUTER_BOUND ( 'NONE', #10754, .T. ) ;
#19932=DIRECTION ( 'NONE',  ( -0.000000000000000000, -0.000000000000000000, 1.000000000000000000 ) ) ;
#19945=DIRECTION ( 'NONE',  ( 0.000000000000000000, 0.000000000000000000, -1.000000000000000000 ) ) ;
#19961=VECTOR ( 'NONE', #55580, 1000.000000000000000 ) ;
#19983=LINE ( 'NONE', #36155, #58793 ) ;
#19984=ORIENTED_EDGE ( 'NONE', *, *, #6077, .T. ) ;
#19989=DIRECTION ( 'NONE',  ( 1.000000000000000000, -0.000000000000000000, 0.000000000000000000 ) ) ;
#19991=ORIENTED_EDGE ( 'NONE', *, *, #64631, .F. ) ;
#19999=DIRECTION ( 'NONE',  ( -0.000000000000000000, -0.000000000000000000, -1.000000000000000000 ) ) ;
#20004=ORIENTED_EDGE ( 'NONE', *, *, #28054, .F. ) ;
#20035=CARTESIAN_POINT ( 'NONE',  ( 0.000000000000000000, 0.000000000000000000, 0.000000000000000000 ) ) ;
#20050=EDGE_LOOP ( 'NONE', ( #58875, #59954, #34918, #17402 ) ) ;
#20075=VERTEX_POINT ( 'NONE', #22527 ) ;
#20080=CARTESIAN_POINT ( 'NONE',  ( 264.4165763529819628, 225.8585178651493948, 138.9999999999999716 ) ) ;
#20096=LINE ( 'NONE', #67950, #2887 ) ;
#20134=FACE_OUTER_BOUND ( 'NONE', #34376, .T. ) ;
#20168=EDGE_CURVE ( 'NONE', #20075, #40730, #24281, .T. ) ;
#20178=CARTESIAN_POINT ( 'NONE',  ( -17.50000000000002842, 207.5000000000000284, 378.0000000000000000 ) ) ;
#20179=CARTESIAN_POINT ( 'NONE',  ( 311.9975424824652350, 295.8720703627916464, 535.5371946177799600 ) ) ;
#20185=DIRECTION ( 'NONE',  ( 0.000000000000000000, 1.000000000000000000, 0.000000000000000000 ) ) ;
#20200=DIRECTION ( 'NONE',  ( 0.000000000000000000, -1.000000000000000000, 0.000000000000000000 ) ) ;
#20213=DIRECTION ( 'NONE',  ( -0.000000000000000000, -0.000000000000000000, -1.000000000000000000 ) ) ;
#20220=ORIENTED_EDGE ( 'NONE', *, *, #61365, .T. ) ;
#20279=CARTESIAN_POINT ( 'NONE',  ( 254.4165763529819344, -27.00000000000000355, 128.9999999999999716 ) ) ;
#20283=DIRECTION ( 'NONE',  ( -1.000000000000000000, 0.000000000000000000, 0.000000000000000000 ) ) ;
#20300=CARTESIAN_POINT ( 'NONE',  ( 111.9975424824652634, 172.0000000000000284, 536.6193948016162949 ) ) ;
#20311=AXIS2_PLACEMENT_3D ( 'NONE', #5406, #65188, #11713 ) ;
#20371=ORIENTED_EDGE ( 'NONE', *, *, #55486, .T. ) ;
#20387=EDGE_CURVE ( 'NONE', #27523, #68787, #38985, .T. ) ;
#20418=EDGE_LOOP ( 'NONE', ( #25518, #324, #28874, #25819 ) ) ;
#20488=ORIENTED_EDGE ( 'NONE', *, *, #21051, .T. ) ;
#20507=ORIENTED_EDGE ( 'NONE', *, *, #11642, .F. ) ;
#20529=EDGE_CURVE ( 'NONE', #4522, #58728, #59717, .T. ) ;
#20540=AXIS2_PLACEMENT_3D ( 'NONE', #63404, #15207, #36669 ) ;
#20596=ORIENTED_EDGE ( 'NONE', *, *, #32094, .F. ) ;
#20626=VERTEX_POINT ( 'NONE', #47025 ) ;
#20661=DIRECTION ( 'NONE',  ( 0.000000000000000000, 0.000000000000000000, 1.000000000000000000 ) ) ;
#20693=DIRECTION ( 'NONE',  ( 1.000000000000000000, 0.000000000000000000, -2.220446049250313081E-16 ) ) ;
#20705=EDGE_CURVE ( 'NONE', #2210, #37473, #34853, .T. ) ;
#20708=ORIENTED_EDGE ( 'NONE', *, *, #5773, .F. ) ;
#20730=CARTESIAN_POINT ( 'NONE',  ( 230.9999999999999432, -57.00000000000007816, -2.000000000000000000 ) ) ;
#20748=CARTESIAN_POINT ( 'NONE',  ( 154.4165763529819628, 225.8585178651493663, 129.0000000000000000 ) ) ;
#20753=CARTESIAN_POINT ( 'NONE',  ( 209.3223706822284100, 0.000000000000000000, 277.8007638641562380 ) ) ;
#20764=DIRECTION ( 'NONE',  ( 1.000000000000000000, 0.000000000000000000, 0.000000000000000000 ) ) ;
#20797=CIRCLE ( 'NONE', #36576, 245.3095347406803342 ) ;
#20810=VERTEX_POINT ( 'NONE', #22109 ) ;
#20816=CARTESIAN_POINT ( 'NONE',  ( 154.4165763529819628, 225.8585178651493663, 108.9999999999999858 ) ) ;
#20822=DIRECTION ( 'NONE',  ( 0.000000000000000000, 0.000000000000000000, 1.000000000000000000 ) ) ;
#20833=CARTESIAN_POINT ( 'NONE',  ( 209.9999999999999716, -57.00000000000007816, 93.99999999999998579 ) ) ;
#20842=CARTESIAN_POINT ( 'NONE',  ( 444.9999999999999432, -35.00000000000000000, -2.000000000000000000 ) ) ;
#20862=DIRECTION ( 'NONE',  ( -1.000000000000000000, 0.000000000000000000, 0.000000000000000000 ) ) ;
#20870=EDGE_CURVE ( 'NONE', #69450, #12534, #37360, .T. ) ;
#20881=ADVANCED_FACE ( 'NONE', ( #53409 ), #59388, .T. ) ;
#20888=CARTESIAN_POINT ( 'NONE',  ( -2.000000000000000000, 0.000000000000000000, -0.000000000000000000 ) ) ;
#20901=VERTEX_POINT ( 'NONE', #44560 ) ;
#20904=CARTESIAN_POINT ( 'NONE',  ( 307.2575771313985342, 170.0000000000000284, 256.6193948016162381 ) ) ;
#20923=ORIENTED_EDGE ( 'NONE', *, *, #18535, .T. ) ;
#21000=LINE ( 'NONE', #10430, #34027 ) ;
#21022=ORIENTED_EDGE ( 'NONE', *, *, #50010, .T. ) ;
#21023=LINE ( 'NONE', #54748, #58950 ) ;
#21045=EDGE_CURVE ( 'NONE', #7345, #32729, #28428, .T. ) ;
#21051=EDGE_CURVE ( 'NONE', #9638, #29599, #12607, .T. ) ;
#21086=CARTESIAN_POINT ( 'NONE',  ( 209.3223706822284100, 0.000000000000000000, 31.44247402469554942 ) ) ;
#21095=ORIENTED_EDGE ( 'NONE', *, *, #4372, .F. ) ;
#21109=DIRECTION ( 'NONE',  ( -1.000000000000000000, 0.000000000000000000, 0.000000000000000000 ) ) ;
#21110=ORIENTED_EDGE ( 'NONE', *, *, #63250, .F. ) ;
#21115=DIRECTION ( 'NONE',  ( 1.000000000000000000, -0.000000000000000000, -0.000000000000000000 ) ) ;
#21162=DIRECTION ( 'NONE',  ( -0.8496664383351307803, 0.000000000000000000, 0.5273205320930463014 ) ) ;
#21184=CARTESIAN_POINT ( 'NONE',  ( 230.9999999999999432, -2.000000000000001776, 72.99999999999998579 ) ) ;
#21196=EDGE_CURVE ( 'NONE', #14640, #37433, #68495, .T. ) ;
#21208=EDGE_CURVE ( 'NONE', #50651, #43728, #42978, .T. ) ;
#21213=LINE ( 'NONE', #63082, #61616 ) ;
#21242=EDGE_LOOP ( 'NONE', ( #6841, #44152, #19143, #19873, #19514, #60481, #47390, #24560, #20488 ) ) ;
#21256=CARTESIAN_POINT ( 'NONE',  ( 0.000000000000000000, 0.000000000000000000, 380.0000000000000000 ) ) ;
#21265=EDGE_CURVE ( 'NONE', #63094, #69498, #11462, .T. ) ;
#21266=ORIENTED_EDGE ( 'NONE', *, *, #21265, .F. ) ;
#21297=DIRECTION ( 'NONE',  ( 0.000000000000000000, 0.000000000000000000, -1.000000000000000000 ) ) ;
#21304=LINE ( 'NONE', #37478, #9526 ) ;
#21341=ORIENTED_EDGE ( 'NONE', *, *, #28865, .T. ) ;
#21372=EDGE_CURVE ( 'NONE', #67311, #47553, #21000, .T. ) ;
#21385=CYLINDRICAL_SURFACE ( 'NONE', #53308, 246.3582898394607241 ) ;
#21402=ADVANCED_FACE ( 'NONE', ( #31551 ), #10778, .T. ) ;
#21412=VECTOR ( 'NONE', #50867, 1000.000000000000000 ) ;
#21425=ORIENTED_EDGE ( 'NONE', *, *, #67351, .T. ) ;
#21443=CARTESIAN_POINT ( 'NONE',  ( 109.9975424824652634, 171.8183490441642221, 533.9018882243740336 ) ) ;
#21455=CIRCLE ( 'NONE', #63033, 5.000000000000004441 ) ;
#21467=VECTOR ( 'NONE', #1804, 1000.000000000000000 ) ;
#21479=DIRECTION ( 'NONE',  ( 0.000000000000000000, 0.000000000000000000, -1.000000000000000000 ) ) ;
#21480=ADVANCED_FACE ( 'NONE', ( #60368 ), #17812, .F. ) ;
#21488=ORIENTED_EDGE ( 'NONE', *, *, #5770, .T. ) ;
#21495=CARTESIAN_POINT ( 'NONE',  ( 410.0000000000000000, 190.0000000000000000, 380.0000000000000000 ) ) ;
#21499=EDGE_CURVE ( 'NONE', #16122, #25612, #54728, .T. ) ;
#21510=EDGE_LOOP ( 'NONE', ( #30673, #53406, #47090, #18727 ) ) ;
#21528=VERTEX_POINT ( 'NONE', #1987 ) ;
#21551=ORIENTED_EDGE ( 'NONE', *, *, #63129, .T. ) ;
#21633=VERTEX_POINT ( 'NONE', #57176 ) ;
#21634=LINE ( 'NONE', #43083, #29135 ) ;
#21637=ORIENTED_EDGE ( 'NONE', *, *, #36373, .F. ) ;
#21641=CARTESIAN_POINT ( 'NONE',  ( 266.9165763529819628, 242.0000000000000000, 128.9999999999999716 ) ) ;
#21674=ADVANCED_FACE ( 'NONE', ( #3363 ), #36065, .F. ) ;
#21678=DIRECTION ( 'NONE',  ( 7.727811381450903769E-14, 0.000000000000000000, 1.000000000000000000 ) ) ;
#21704=CIRCLE ( 'NONE', #30713, 245.3095347406802489 ) ;
#21720=LINE ( 'NONE', #64644, #21750 ) ;
#21750=VECTOR ( 'NONE', #1662, 1000.000000000000000 ) ;
#21755=VERTEX_POINT ( 'NONE', #38476 ) ;
#21768=ORIENTED_EDGE ( 'NONE', *, *, #64022, .F. ) ;
#21809=DIRECTION ( 'NONE',  ( 0.000000000000000000, -0.000000000000000000, -1.000000000000000000 ) ) ;
#21820=EDGE_CURVE ( 'NONE', #31511, #61512, #33212, .T. ) ;
#21824=CARTESIAN_POINT ( 'NONE',  ( 188.9999999999999432, 190.0000000000000000, 72.99999999999998579 ) ) ;
#21841=CIRCLE ( 'NONE', #62283, 5.000000000000000888 ) ;
#21904=ORIENTED_EDGE ( 'NONE', *, *, #16359, .T. ) ;
#21914=FACE_OUTER_BOUND ( 'NONE', #35253, .T. ) ;
#21931=ADVANCED_FACE ( 'NONE', ( #39702 ), #56570, .F. ) ;
#21936=ORIENTED_EDGE ( 'NONE', *, *, #29449, .F. ) ;
#21942=AXIS2_PLACEMENT_3D ( 'NONE', #32846, #6106, #55340 ) ;
#21969=CARTESIAN_POINT ( 'NONE',  ( 427.4999999999999432, 207.5000000000000284, 0.000000000000000000 ) ) ;
#21993=PLANE ( 'NONE',  #23363 ) ;
#22014=VERTEX_POINT ( 'NONE', #61506 ) ;
#22026=EDGE_LOOP ( 'NONE', ( #8794, #36712 ) ) ;
#22042=LINE ( 'NONE', #32600, #24025 ) ;
#22044=CARTESIAN_POINT ( 'NONE',  ( -35.00000000000002842, -35.00000000000000000, 380.0000000000000000 ) ) ;
#22052=ORIENTED_EDGE ( 'NONE', *, *, #13376, .F. ) ;
#22055=LINE ( 'NONE', #2012, #38515 ) ;
#22108=VERTEX_POINT ( 'NONE', #52664 ) ;
#22109=CARTESIAN_POINT ( 'NONE',  ( 188.9999999999999432, 192.0000000000000000, 0.000000000000000000 ) ) ;
#22134=CARTESIAN_POINT ( 'NONE',  ( 209.9518228411288874, 172.0000000000000284, 31.43423095485942298 ) ) ;
#22151=VERTEX_POINT ( 'NONE', #24579 ) ;
#22152=CARTESIAN_POINT ( 'NONE',  ( 266.9165763529819628, -52.00000000000000711, 128.9999999999999716 ) ) ;
#22175=ORIENTED_EDGE ( 'NONE', *, *, #60985, .T. ) ;
#22195=ORIENTED_EDGE ( 'NONE', *, *, #28849, .F. ) ;
#22205=LINE ( 'NONE', #43292, #64007 ) ;
#22210=ORIENTED_EDGE ( 'NONE', *, *, #41691, .T. ) ;
#22211=AXIS2_PLACEMENT_3D ( 'NONE', #58274, #63904, #26276 ) ;
#22236=CIRCLE ( 'NONE', #59278, 5.000000000000004441 ) ;
#22264=ORIENTED_EDGE ( 'NONE', *, *, #39272, .F. ) ;
#22332=EDGE_CURVE ( 'NONE', #30991, #28403, #34359, .T. ) ;
#22356=LINE ( 'NONE', #37840, #49389 ) ;
#22362=VERTEX_POINT ( 'NONE', #17456 ) ;
#22486=CARTESIAN_POINT ( 'NONE',  ( 412.0000000000000000, 192.0000000000000000, 380.0000000000000000 ) ) ;
#22503=DIRECTION ( 'NONE',  ( -0.000000000000000000, -0.000000000000000000, -1.000000000000000000 ) ) ;
#22506=ORIENTED_EDGE ( 'NONE', *, *, #51233, .T. ) ;
#22509=ORIENTED_EDGE ( 'NONE', *, *, #9143, .F. ) ;
#22527=CARTESIAN_POINT ( 'NONE',  ( 188.9999999999999432, -35.00000000000000000, 0.000000000000000000 ) ) ;
#22530=EDGE_CURVE ( 'NONE', #42281, #45595, #5771, .T. ) ;
#22531=CARTESIAN_POINT ( 'NONE',  ( -17.50000000000002842, -18.06806526123148160, 0.000000000000000000 ) ) ;
#22541=ORIENTED_EDGE ( 'NONE', *, *, #15413, .T. ) ;
#22600=ORIENTED_EDGE ( 'NONE', *, *, #29018, .F. ) ;
#22613=AXIS2_PLACEMENT_3D ( 'NONE', #3743, #19932, #40338 ) ;
#22622=DIRECTION ( 'NONE',  ( 0.000000000000000000, -0.000000000000000000, -1.000000000000000000 ) ) ;
#22626=ORIENTED_EDGE ( 'NONE', *, *, #31980, .F. ) ;
#22670=DIRECTION ( 'NONE',  ( -0.000000000000000000, 0.02271222823333339177, -0.9997420440737084801 ) ) ;
#22672=CARTESIAN_POINT ( 'NONE',  ( 209.3223706822284100, 0.000000000000000000, 31.44247402469554942 ) ) ;
#22691=ORIENTED_EDGE ( 'NONE', *, *, #60489, .F. ) ;
#22717=FACE_OUTER_BOUND ( 'NONE', #68381, .T. ) ;
#22759=AXIS2_PLACEMENT_3D ( 'NONE', #50640, #7037, #61549 ) ;
#22766=CARTESIAN_POINT ( 'NONE',  ( 144.4165763529819344, 225.8585178651493663, 108.9999999999999858 ) ) ;
#22771=ADVANCED_FACE ( 'NONE', ( #5360 ), #10974, .F. ) ;
#22809=LINE ( 'NONE', #27730, #52231 ) ;
#22818=VECTOR ( 'NONE', #9794, 1000.000000000000000 ) ;
#22822=VECTOR ( 'NONE', #22670, 1000.000000000000114 ) ;
#22834=CARTESIAN_POINT ( 'NONE',  ( 141.9165763529819344, 242.0000000000000000, 108.9999999999999858 ) ) ;
#22847=CARTESIAN_POINT ( 'NONE',  ( 33.99754248246522792, 18.00000000000002842, 401.6295345748407613 ) ) ;
#22870=CARTESIAN_POINT ( 'NONE',  ( 109.9975424824652777, 296.0000000000000000, 418.0000000000000000 ) ) ;
#22921=VECTOR ( 'NONE', #58364, 1000.000000000000000 ) ;
#22925=CYLINDRICAL_SURFACE ( 'NONE', #35422, 5.000000000000004441 ) ;
#22931=VECTOR ( 'NONE', #2179, 1000.000000000000000 ) ;
#22945=LINE ( 'NONE', #54940, #15571 ) ;
#22954=DIRECTION ( 'NONE',  ( 0.000000000000000000, 0.000000000000000000, 1.000000000000000000 ) ) ;
#23049=EDGE_CURVE ( 'NONE', #17967, #40644, #30637, .T. ) ;
#23074=DIRECTION ( 'NONE',  ( 0.000000000000000000, -1.000000000000000000, -0.000000000000000000 ) ) ;
#23079=CARTESIAN_POINT ( 'NONE',  ( 209.9518228411288874, 172.0000000000000284, 31.43423095485942298 ) ) ;
#23095=LINE ( 'NONE', #34950, #25453 ) ;
#23119=DIRECTION ( 'NONE',  ( -1.000000000000000000, 0.000000000000000000, 0.000000000000000000 ) ) ;
#23131=EDGE_CURVE ( 'NONE', #13211, #58078, #30986, .T. ) ;
#23175=CARTESIAN_POINT ( 'NONE',  ( 141.9165763529819344, -52.00000000000000711, 108.9999999999999858 ) ) ;
#23192=LINE ( 'NONE', #28456, #1680 ) ;
#23218=AXIS2_PLACEMENT_3D ( 'NONE', #42782, #69175, #37512 ) ;
#23305=LINE ( 'NONE', #18017, #43983 ) ;
#23354=ORIENTED_EDGE ( 'NONE', *, *, #6159, .F. ) ;
#23358=ORIENTED_EDGE ( 'NONE', *, *, #39722, .F. ) ;
#23363=AXIS2_PLACEMENT_3D ( 'NONE', #48699, #16021, #52954 ) ;
#23377=EDGE_CURVE ( 'NONE', #19781, #1198, #21841, .T. ) ;
#23383=ORIENTED_EDGE ( 'NONE', *, *, #38668, .F. ) ;
#23422=AXIS2_PLACEMENT_3D ( 'NONE', #18795, #29022, #2974 ) ;
#23430=FACE_OUTER_BOUND ( 'NONE', #55710, .T. ) ;
#23444=DIRECTION ( 'NONE',  ( -1.000000000000000000, -0.000000000000000000, -0.000000000000000000 ) ) ;
#23452=ORIENTED_EDGE ( 'NONE', *, *, #4527, .T. ) ;
#23461=CARTESIAN_POINT ( 'NONE',  ( -35.00000000000002842, -35.00000000000000000, -2.000000000000000000 ) ) ;
#23481=ORIENTED_EDGE ( 'NONE', *, *, #69148, .F. ) ;
#23494=CARTESIAN_POINT ( 'NONE',  ( -35.00000000000002842, -35.00000000000000000, -2.000000000000000000 ) ) ;
#23523=CARTESIAN_POINT ( 'NONE',  ( 109.9975424824652634, 172.0000000000000284, 256.8908838121927261 ) ) ;
#23534=CARTESIAN_POINT ( 'NONE',  ( -22.50000000000003197, -18.06806526123148160, 378.0000000000000000 ) ) ;
#23540=CARTESIAN_POINT ( 'NONE',  ( 0.000000000000000000, 190.0000000000000000, 380.0000000000000000 ) ) ;
#23541=ORIENTED_EDGE ( 'NONE', *, *, #20870, .F. ) ;
#23548=ORIENTED_EDGE ( 'NONE', *, *, #63250, .T. ) ;
#23553=ORIENTED_EDGE ( 'NONE', *, *, #9143, .T. ) ;
#23562=DIRECTION ( 'NONE',  ( 0.000000000000000000, 0.000000000000000000, -1.000000000000000000 ) ) ;
#23570=VECTOR ( 'NONE', #65970, 1000.000000000000000 ) ;
#23599=EDGE_CURVE ( 'NONE', #2210, #14720, #2430, .T. ) ;
#23648=VECTOR ( 'NONE', #28367, 1000.000000000000000 ) ;
#23656=EDGE_CURVE ( 'NONE', #4597, #46092, #44985, .T. ) ;
#23666=ORIENTED_EDGE ( 'NONE', *, *, #43959, .T. ) ;
#23672=ADVANCED_FACE ( 'NONE', ( #61519 ), #55535, .F. ) ;
#23692=ORIENTED_EDGE ( 'NONE', *, *, #17292, .T. ) ;
#23702=EDGE_CURVE ( 'NONE', #62233, #7559, #40746, .T. ) ;
#23726=DIRECTION ( 'NONE',  ( -0.000000000000000000, -0.000000000000000000, -1.000000000000000000 ) ) ;
#23752=EDGE_CURVE ( 'NONE', #54755, #69128, #12996, .T. ) ;
#23759=EDGE_CURVE ( 'NONE', #47060, #17967, #14033, .T. ) ;
#23769=DIRECTION ( 'NONE',  ( 0.000000000000000000, 1.000000000000000000, -0.000000000000000000 ) ) ;
#23770=LINE ( 'NONE', #28341, #19653 ) ;
#23773=EDGE_LOOP ( 'NONE', ( #11955, #66661, #29373, #21904 ) ) ;
#23788=ORIENTED_EDGE ( 'NONE', *, *, #43792, .T. ) ;
#23849=PLANE ( 'NONE',  #67912 ) ;
#23853=EDGE_LOOP ( 'NONE', ( #2043, #51818, #36277, #32118 ) ) ;
#23868=ORIENTED_EDGE ( 'NONE', *, *, #32572, .F. ) ;
#23889=CARTESIAN_POINT ( 'NONE',  ( 0.000000000000000000, -1.426547569622074412E-15, 159.3522585083728131 ) ) ;
#23894=EDGE_LOOP ( 'NONE', ( #45647, #39948, #3182, #56900 ) ) ;
#23915=DIRECTION ( 'NONE',  ( 0.000000000000000000, 0.000000000000000000, 1.000000000000000000 ) ) ;
#23927=VERTEX_POINT ( 'NONE', #50184 ) ;
#23934=VECTOR ( 'NONE', #10288, 1000.000000000000000 ) ;
#23982=VECTOR ( 'NONE', #26515, 1000.000000000000000 ) ;
#23997=CARTESIAN_POINT ( 'NONE',  ( 188.9999999999999432, -35.00000000000000000, -2.000000000000000888 ) ) ;
#24020=DIRECTION ( 'NONE',  ( -1.000000000000000000, 0.000000000000000000, 0.000000000000000000 ) ) ;
#24021=LINE ( 'NONE', #3947, #51154 ) ;
#24025=VECTOR ( 'NONE', #17097, 1000.000000000000000 ) ;
#24045=DIRECTION ( 'NONE',  ( -1.000000000000000000, 0.000000000000000000, 0.000000000000000000 ) ) ;
#24063=EDGE_LOOP ( 'NONE', ( #7606, #18381, #46614, #20220, #27705, #44645 ) ) ;
#24068=DIRECTION ( 'NONE',  ( -0.000000000000000000, 1.000000000000000000, -0.000000000000000000 ) ) ;
#24118=CARTESIAN_POINT ( 'NONE',  ( 109.9975424824652634, 179.2896996249788799, 369.5505932007772003 ) ) ;
#24143=AXIS2_PLACEMENT_3D ( 'NONE', #41018, #29768, #68440 ) ;
#24152=DIRECTION ( 'NONE',  ( 0.000000000000000000, 1.000000000000000000, -0.000000000000000000 ) ) ;
#24168=LINE ( 'NONE', #40672, #46956 ) ;
#24171=ORIENTED_EDGE ( 'NONE', *, *, #40114, .F. ) ;
#24178=ORIENTED_EDGE ( 'NONE', *, *, #314, .F. ) ;
#24224=VECTOR ( 'NONE', #27639, 1000.000000000000000 ) ;
#24226=EDGE_CURVE ( 'NONE', #8357, #11118, #2963, .T. ) ;
#24232=CARTESIAN_POINT ( 'NONE',  ( 141.9165763529819344, -52.00000000000000711, 129.0000000000000000 ) ) ;
#24279=DIRECTION ( 'NONE',  ( 0.000000000000000000, 0.000000000000000000, -1.000000000000000000 ) ) ;
#24281=LINE ( 'NONE', #51008, #57522 ) ;
#24282=VECTOR ( 'NONE', #19999, 1000.000000000000000 ) ;
#24287=VECTOR ( 'NONE', #35264, 1000.000000000000000 ) ;
#24288=CARTESIAN_POINT ( 'NONE',  ( 230.9999999999999432, 192.0000000000000000, 380.0000000000000000 ) ) ;
#24366=EDGE_LOOP ( 'NONE', ( #52374, #22691, #49672, #40852, #8031, #28977 ) ) ;
#24415=EDGE_CURVE ( 'NONE', #60658, #42281, #30856, .T. ) ;
#24456=ORIENTED_EDGE ( 'NONE', *, *, #45675, .T. ) ;
#24472=EDGE_CURVE ( 'NONE', #52352, #58078, #28920, .T. ) ;
#24485=DIRECTION ( 'NONE',  ( 0.000000000000000000, 0.000000000000000000, -1.000000000000000000 ) ) ;
#24528=AXIS2_PLACEMENT_3D ( 'NONE', #22152, #64359, #37630 ) ;
#24548=CARTESIAN_POINT ( 'NONE',  ( -22.50000000000003197, -18.06806526123148160, 380.0000000000000000 ) ) ;
#24560=ORIENTED_EDGE ( 'NONE', *, *, #54151, .T. ) ;
#24579=CARTESIAN_POINT ( 'NONE',  ( 111.9975424824652634, 296.0000000000000000, 529.9060149868646477 ) ) ;
#24593=CARTESIAN_POINT ( 'NONE',  ( 311.9975424824652350, 170.0000000000000284, 536.6193948016162949 ) ) ;
#24616=CARTESIAN_POINT ( 'NONE',  ( 0.000000000000000000, 0.000000000000000000, 380.0000000000000000 ) ) ;
#24631=ORIENTED_EDGE ( 'NONE', *, *, #43171, .F. ) ;
#24655=ORIENTED_EDGE ( 'NONE', *, *, #25346, .F. ) ;
#24672=CARTESIAN_POINT ( 'NONE',  ( 432.4999999999999432, 207.5000000000000284, 378.0000000000000000 ) ) ;
#24679=AXIS2_PLACEMENT_3D ( 'NONE', #4435, #53638, #21297 ) ;
#24730=DIRECTION ( 'NONE',  ( -0.000000000000000000, 1.000000000000000000, 0.000000000000000000 ) ) ;
#24768=LINE ( 'NONE', #39559, #63084 ) ;
#24774=CARTESIAN_POINT ( 'NONE',  ( 0.000000000000000000, 192.0000000000000000, 0.000000000000000000 ) ) ;
#24781=CARTESIAN_POINT ( 'NONE',  ( 311.9975424824652350, 170.0000000000000284, 254.5114349394235091 ) ) ;
#24844=CARTESIAN_POINT ( 'NONE',  ( -17.50000000000002842, 207.5000000000000284, 0.000000000000000000 ) ) ;
#24852=DIRECTION ( 'NONE',  ( -0.000000000000000000, -0.000000000000000000, 1.000000000000000000 ) ) ;
#24892=CIRCLE ( 'NONE', #63095, 5.000000000000004441 ) ;
#24965=VERTEX_POINT ( 'NONE', #39905 ) ;
#24968=DIRECTION ( 'NONE',  ( 0.000000000000000000, 0.000000000000000000, -1.000000000000000000 ) ) ;
#24970=CARTESIAN_POINT ( 'NONE',  ( -12.50000000000002842, -18.06806526123148160, 378.0000000000000000 ) ) ;
#24971=CARTESIAN_POINT ( 'NONE',  ( 230.9999999999999432, -57.00000000000007816, -2.000000000000000000 ) ) ;
#24989=AXIS2_PLACEMENT_3D ( 'NONE', #3486, #3157, #57992 ) ;
#24998=CIRCLE ( 'NONE', #55301, 246.3582898394607525 ) ;
#25002=FACE_OUTER_BOUND ( 'NONE', #18266, .T. ) ;
#25033=ORIENTED_EDGE ( 'NONE', *, *, #31787, .T. ) ;
#25072=DIRECTION ( 'NONE',  ( 1.000000000000000000, 0.000000000000000000, 0.000000000000000000 ) ) ;
#25094=CARTESIAN_POINT ( 'NONE',  ( 311.9975424824652350, 170.0000000000000284, 380.0000000000001137 ) ) ;
#25101=DIRECTION ( 'NONE',  ( 0.000000000000000000, 1.000000000000000000, 0.000000000000000000 ) ) ;
#25126=PLANE ( 'NONE',  #31254 ) ;
#25132=ORIENTED_EDGE ( 'NONE', *, *, #41862, .F. ) ;
#25160=ORIENTED_EDGE ( 'NONE', *, *, #54935, .F. ) ;
#25172=PLANE ( 'NONE',  #2831 ) ;
#25174=DIRECTION ( 'NONE',  ( 0.000000000000000000, 0.000000000000000000, 1.000000000000000000 ) ) ;
#25184=CARTESIAN_POINT ( 'NONE',  ( -12.50000000000002842, 207.5000000000000284, -2.000000000000000000 ) ) ;
#25214=VERTEX_POINT ( 'NONE', #46207 ) ;
#25218=ORIENTED_EDGE ( 'NONE', *, *, #50991, .T. ) ;
#25245=VECTOR ( 'NONE', #30754, 1000.000000000000000 ) ;
#25272=LINE ( 'NONE', #68185, #5273 ) ;
#25303=CARTESIAN_POINT ( 'NONE',  ( 188.9999999999999432, -2.000000000000001776, 72.99999999999998579 ) ) ;
#25323=EDGE_LOOP ( 'NONE', ( #24171, #21768, #25033, #65250 ) ) ;
#25346=EDGE_CURVE ( 'NONE', #58728, #2957, #58481, .T. ) ;
#25386=ORIENTED_EDGE ( 'NONE', *, *, #1020, .F. ) ;
#25425=EDGE_CURVE ( 'NONE', #21633, #39050, #47926, .T. ) ;
#25437=ORIENTED_EDGE ( 'NONE', *, *, #52443, .T. ) ;
#25438=ADVANCED_FACE ( 'NONE', ( #2535 ), #44034, .F. ) ;
#25443=DIRECTION ( 'NONE',  ( -0.000000000000000000, 1.000000000000000000, -0.000000000000000000 ) ) ;
#25453=VECTOR ( 'NONE', #44543, 1000.000000000000000 ) ;
#25473=FACE_BOUND ( 'NONE', #27153, .T. ) ;
#25503=DIRECTION ( 'NONE',  ( 0.000000000000000000, 0.000000000000000000, 1.000000000000000000 ) ) ;
#25509=DIRECTION ( 'NONE',  ( -0.000000000000000000, 0.000000000000000000, -1.000000000000000000 ) ) ;
#25518=ORIENTED_EDGE ( 'NONE', *, *, #48997, .F. ) ;
#25542=VECTOR ( 'NONE', #33738, 1000.000000000000000 ) ;
#25562=DIRECTION ( 'NONE',  ( -1.000000000000000000, 0.000000000000000000, 0.000000000000000000 ) ) ;
#25568=DIRECTION ( 'NONE',  ( 1.000000000000000000, 0.000000000000000000, -2.220446049250313081E-16 ) ) ;
#25580=EDGE_CURVE ( 'NONE', #13843, #33368, #20096, .T. ) ;
#25602=CARTESIAN_POINT ( 'NONE',  ( 149.4165763529819344, -26.99999999999998224, 108.9999999999999858 ) ) ;
#25612=VERTEX_POINT ( 'NONE', #68623 ) ;
#25649=AXIS2_PLACEMENT_3D ( 'NONE', #26881, #65569, #54646 ) ;
#25666=DIRECTION ( 'NONE',  ( 1.000000000000000000, 0.000000000000000000, -0.000000000000000000 ) ) ;
#25684=EDGE_LOOP ( 'NONE', ( #17308, #34791, #31778, #22052, #46432, #17710, #62604, #16695, #44227, #20708, #64791 ) ) ;
#25751=DIRECTION ( 'NONE',  ( 0.000000000000000000, 0.000000000000000000, 1.000000000000000000 ) ) ;
#25780=VECTOR ( 'NONE', #50037, 1000.000000000000000 ) ;
#25807=ORIENTED_EDGE ( 'NONE', *, *, #50010, .F. ) ;
#25817=ADVANCED_FACE ( 'NONE', ( #53806 ), #64374, .T. ) ;
#25819=ORIENTED_EDGE ( 'NONE', *, *, #56960, .T. ) ;
#25852=DIRECTION ( 'NONE',  ( -0.000000000000000000, 0.000000000000000000, 1.000000000000000000 ) ) ;
#25895=ORIENTED_EDGE ( 'NONE', *, *, #59468, .T. ) ;
#25904=FACE_OUTER_BOUND ( 'NONE', #62998, .T. ) ;
#25915=ORIENTED_EDGE ( 'NONE', *, *, #54213, .F. ) ;
#25943=ORIENTED_EDGE ( 'NONE', *, *, #22332, .F. ) ;
#25963=CARTESIAN_POINT ( 'NONE',  ( 259.4165763529819060, 225.8585178651493948, 128.9999999999999716 ) ) ;
#25966=ADVANCED_FACE ( 'NONE', ( #32302 ), #21385, .T. ) ;
#25993=AXIS2_PLACEMENT_3D ( 'NONE', #13856, #55735, #56778 ) ;
#26028=ORIENTED_EDGE ( 'NONE', *, *, #59785, .F. ) ;
#26034=CARTESIAN_POINT ( 'NONE',  ( 409.0783954480987177, 190.0000000000000000, 174.7010307253932808 ) ) ;
#26045=ADVANCED_FACE ( 'NONE', ( #9286 ), #51850, .T. ) ;
#26072=CARTESIAN_POINT ( 'NONE',  ( 427.4999999999999432, 207.5000000000000284, 378.0000000000000000 ) ) ;
#26083=EDGE_LOOP ( 'NONE', ( #575, #21551 ) ) ;
#26090=VERTEX_POINT ( 'NONE', #19847 ) ;
#26166=VERTEX_POINT ( 'NONE', #16627 ) ;
#26187=DIRECTION ( 'NONE',  ( -0.000000000000000000, -0.000000000000000000, -1.000000000000000000 ) ) ;
#26194=DIRECTION ( 'NONE',  ( 0.000000000000000000, 1.000000000000000000, 0.000000000000000000 ) ) ;
#26204=ORIENTED_EDGE ( 'NONE', *, *, #4439, .F. ) ;
#26209=CARTESIAN_POINT ( 'NONE',  ( 111.9975424824652634, 295.8720703627916464, 535.5371946177799600 ) ) ;
#26235=ORIENTED_EDGE ( 'NONE', *, *, #38259, .T. ) ;
#26247=PLANE ( 'NONE',  #37354 ) ;
#26255=VERTEX_POINT ( 'NONE', #43001 ) ;
#26276=DIRECTION ( 'NONE',  ( -1.000000000000000000, 0.000000000000000000, 0.000000000000000000 ) ) ;
#26277=DIRECTION ( 'NONE',  ( 0.000000000000000000, -1.000000000000000000, 0.000000000000000000 ) ) ;
#26417=DIRECTION ( 'NONE',  ( 1.000000000000000000, 0.000000000000000000, 0.000000000000000000 ) ) ;
#26418=ORIENTED_EDGE ( 'NONE', *, *, #53401, .F. ) ;
#26419=FACE_BOUND ( 'NONE', #53781, .T. ) ;
#26456=ORIENTED_EDGE ( 'NONE', *, *, #41862, .T. ) ;
#26471=VECTOR ( 'NONE', #27986, 1000.000000000000000 ) ;
#26515=DIRECTION ( 'NONE',  ( 1.000000000000000000, 0.000000000000000000, 0.000000000000000000 ) ) ;
#26549=EDGE_LOOP ( 'NONE', ( #13148, #43088 ) ) ;
#26558=CARTESIAN_POINT ( 'NONE',  ( 410.0000000000000000, 190.0000000000000000, 175.2157797990580832 ) ) ;
#26568=VECTOR ( 'NONE', #29247, 1000.000000000000000 ) ;
#26587=DIRECTION ( 'NONE',  ( -1.000000000000000000, -0.000000000000000000, -0.000000000000000000 ) ) ;
#26645=CARTESIAN_POINT ( 'NONE',  ( 209.9999999999999716, 190.0000000000000000, 93.99999999999998579 ) ) ;
#26675=AXIS2_PLACEMENT_3D ( 'NONE', #29286, #51445, #25751 ) ;
#26676=EDGE_LOOP ( 'NONE', ( #37774, #69182 ) ) ;
#26678=EDGE_CURVE ( 'NONE', #49819, #54192, #47880, .T. ) ;
#26689=FACE_OUTER_BOUND ( 'NONE', #11075, .T. ) ;
#26694=PLANE ( 'NONE',  #45448 ) ;
#26728=ORIENTED_EDGE ( 'NONE', *, *, #53903, .T. ) ;
#26777=DIRECTION ( 'NONE',  ( -1.000000000000000000, 0.000000000000000000, 0.000000000000000000 ) ) ;
#26811=DIRECTION ( 'NONE',  ( 0.000000000000000000, 1.000000000000000000, -0.000000000000000000 ) ) ;
#26837=CARTESIAN_POINT ( 'NONE',  ( 313.9975424824652350, 295.8720703627917601, 535.5371946177799600 ) ) ;
#26858=CARTESIAN_POINT ( 'NONE',  ( -35.00000000000002842, -35.00000000000000000, 380.0000000000000000 ) ) ;
#26881=CARTESIAN_POINT ( 'NONE',  ( 149.4165763529819344, 225.8585178651493663, 129.0000000000000000 ) ) ;
#26906=EDGE_CURVE ( 'NONE', #67175, #61739, #8461, .T. ) ;
#26907=ORIENTED_EDGE ( 'NONE', *, *, #52948, .T. ) ;
#26920=ORIENTED_EDGE ( 'NONE', *, *, #21820, .T. ) ;
#26928=CARTESIAN_POINT ( 'NONE',  ( 111.9975424824652634, 170.0000000000000284, 354.1673509436691347 ) ) ;
#26943=VECTOR ( 'NONE', #33019, 1000.000000000000000 ) ;
#27005=PLANE ( 'NONE',  #40125 ) ;
#27013=FACE_OUTER_BOUND ( 'NONE', #56550, .T. ) ;
#27041=EDGE_CURVE ( 'NONE', #7559, #36317, #22809, .T. ) ;
#27042=CARTESIAN_POINT ( 'NONE',  ( 111.9975424824652634, 20.00000000000003197, 536.6193948016162949 ) ) ;
#27052=CYLINDRICAL_SURFACE ( 'NONE', #2999, 5.000000000000004441 ) ;
#27059=EDGE_CURVE ( 'NONE', #4597, #295, #42858, .T. ) ;
#27066=ORIENTED_EDGE ( 'NONE', *, *, #42498, .T. ) ;
#27073=AXIS2_PLACEMENT_3D ( 'NONE', #1493, #33523, #22954 ) ;
#27093=ADVANCED_FACE ( 'NONE', ( #3696 ), #25172, .F. ) ;
#27144=ORIENTED_EDGE ( 'NONE', *, *, #32916, .T. ) ;
#27153=EDGE_LOOP ( 'NONE', ( #8837, #18090 ) ) ;
#27191=CARTESIAN_POINT ( 'NONE',  ( 209.9999999999999716, -2.000000000000001776, 72.99999999999998579 ) ) ;
#27216=CIRCLE ( 'NONE', #66569, 5.000000000000004441 ) ;
#27243=FACE_OUTER_BOUND ( 'NONE', #5927, .T. ) ;
#27268=DIRECTION ( 'NONE',  ( 0.000000000000000000, 1.000000000000000000, 0.000000000000000000 ) ) ;
#27288=CARTESIAN_POINT ( 'NONE',  ( 230.9999999999999432, 0.000000000000000000, 380.0000000000000000 ) ) ;
#27290=EDGE_CURVE ( 'NONE', #57264, #45595, #19744, .T. ) ;
#27304=LINE ( 'NONE', #37872, #68906 ) ;
#27306=CARTESIAN_POINT ( 'NONE',  ( 432.4999999999999432, 207.5000000000000284, 378.0000000000000000 ) ) ;
#27318=LINE ( 'NONE', #49110, #9518 ) ;
#27351=DIRECTION ( 'NONE',  ( 0.000000000000000000, 0.000000000000000000, -1.000000000000000000 ) ) ;
#27352=EDGE_LOOP ( 'NONE', ( #16728, #59994, #35474, #19756 ) ) ;
#27376=EDGE_CURVE ( 'NONE', #11698, #57527, #38835, .T. ) ;
#27402=LINE ( 'NONE', #22834, #53274 ) ;
#27429=DIRECTION ( 'NONE',  ( 0.000000000000000000, 0.04541273895899305968, -0.9989683093773508160 ) ) ;
#27457=DIRECTION ( 'NONE',  ( -0.000000000000000000, -0.000000000000000000, -1.000000000000000000 ) ) ;
#27489=ADVANCED_FACE ( 'NONE', ( #29315 ), #66966, .T. ) ;
#27491=VERTEX_POINT ( 'NONE', #18764 ) ;
#27523=VERTEX_POINT ( 'NONE', #51471 ) ;
#27536=CARTESIAN_POINT ( 'NONE',  ( 0.000000000000000000, 0.000000000000000000, 380.0000000000000000 ) ) ;
#27540=DIRECTION ( 'NONE',  ( -0.000000000000000000, -0.000000000000000000, 1.000000000000000000 ) ) ;
#27543=LINE ( 'NONE', #53576, #42791 ) ;
#27546=CARTESIAN_POINT ( 'NONE',  ( 259.4165763529819060, -27.00000000000000355, 138.9999999999999716 ) ) ;
#27553=CARTESIAN_POINT ( 'NONE',  ( 427.4999999999999432, 207.5000000000000284, 378.0000000000000000 ) ) ;
#27612=FACE_OUTER_BOUND ( 'NONE', #9528, .T. ) ;
#27631=EDGE_CURVE ( 'NONE', #8984, #26090, #6383, .T. ) ;
#27633=LINE ( 'NONE', #11796, #42199 ) ;
#27639=DIRECTION ( 'NONE',  ( 1.000000000000000000, 0.000000000000000000, 0.000000000000000000 ) ) ;
#27645=ORIENTED_EDGE ( 'NONE', *, *, #51233, .F. ) ;
#27646=VERTEX_POINT ( 'NONE', #44003 ) ;
#27680=EDGE_LOOP ( 'NONE', ( #62715, #39407, #69125, #13287 ) ) ;
#27684=LINE ( 'NONE', #64989, #36818 ) ;
#27703=ORIENTED_EDGE ( 'NONE', *, *, #60071, .T. ) ;
#27705=ORIENTED_EDGE ( 'NONE', *, *, #11890, .F. ) ;
#27718=CARTESIAN_POINT ( 'NONE',  ( 313.9975424824652350, 179.2896996249788799, 369.5505932007772003 ) ) ;
#27730=CARTESIAN_POINT ( 'NONE',  ( 109.9975424824652777, 172.0000000000000284, 418.0000000000000000 ) ) ;
#27738=ORIENTED_EDGE ( 'NONE', *, *, #37321, .F. ) ;
#27780=CARTESIAN_POINT ( 'NONE',  ( 109.9975424824652634, 18.00000000000002842, 256.8908838121927261 ) ) ;
#27801=EDGE_CURVE ( 'NONE', #26090, #52456, #34320, .T. ) ;
#27809=DIRECTION ( 'NONE',  ( -0.000000000000000000, -0.000000000000000000, -1.000000000000000000 ) ) ;
#27812=DIRECTION ( 'NONE',  ( 0.000000000000000000, 0.000000000000000000, 1.000000000000000000 ) ) ;
#27814=ORIENTED_EDGE ( 'NONE', *, *, #37497, .F. ) ;
#27824=LINE ( 'NONE', #21495, #14338 ) ;
#27834=DIRECTION ( 'NONE',  ( -0.8532989592251507549, 0.000000000000000000, 0.5214219847544545594 ) ) ;
#27840=CARTESIAN_POINT ( 'NONE',  ( 141.9165763529819344, 192.0000000000000000, 108.9999999999999858 ) ) ;
#27890=DIRECTION ( 'NONE',  ( -0.000000000000000000, -0.000000000000000000, -1.000000000000000000 ) ) ;
#27971=CYLINDRICAL_SURFACE ( 'NONE', #34, 5.000000000000004441 ) ;
#27983=ORIENTED_EDGE ( 'NONE', *, *, #32393, .F. ) ;
#27986=DIRECTION ( 'NONE',  ( 0.000000000000000000, 0.000000000000000000, 1.000000000000000000 ) ) ;
#27987=CARTESIAN_POINT ( 'NONE',  ( 149.4165763529819344, 225.8585178651493663, 108.9999999999999858 ) ) ;
#27991=DIRECTION ( 'NONE',  ( 0.000000000000000000, 0.000000000000000000, 1.000000000000000000 ) ) ;
#28012=DIRECTION ( 'NONE',  ( -1.000000000000000000, 0.000000000000000000, -0.000000000000000000 ) ) ;
#28017=DIRECTION ( 'NONE',  ( -0.000000000000000000, 1.000000000000000000, -0.000000000000000000 ) ) ;
#28021=ORIENTED_EDGE ( 'NONE', *, *, #1668, .T. ) ;
#28033=VECTOR ( 'NONE', #9404, 1000.000000000000000 ) ;
#28047=DIRECTION ( 'NONE',  ( -1.000000000000000000, 0.000000000000000000, 0.000000000000000000 ) ) ;
#28054=EDGE_CURVE ( 'NONE', #40156, #20810, #66110, .T. ) ;
#28078=EDGE_CURVE ( 'NONE', #16701, #34756, #7702, .T. ) ;
#28083=DIRECTION ( 'NONE',  ( -1.000000000000000000, 0.000000000000000000, 0.000000000000000000 ) ) ;
#28102=DIRECTION ( 'NONE',  ( 0.000000000000000000, -1.000000000000000000, -0.000000000000000000 ) ) ;
#28112=EDGE_CURVE ( 'NONE', #13050, #36317, #13326, .T. ) ;
#28124=ORIENTED_EDGE ( 'NONE', *, *, #297, .F. ) ;
#28136=ORIENTED_EDGE ( 'NONE', *, *, #39362, .T. ) ;
#28183=CIRCLE ( 'NONE', #1277, 5.000000000000000888 ) ;
#28197=ORIENTED_EDGE ( 'NONE', *, *, #23702, .T. ) ;
#28233=AXIS2_PLACEMENT_3D ( 'NONE', #52472, #9222, #4296 ) ;
#28294=CARTESIAN_POINT ( 'NONE',  ( -17.50000000000002842, -18.06806526123148160, 378.0000000000000000 ) ) ;
#28331=ORIENTED_EDGE ( 'NONE', *, *, #46763, .T. ) ;
#28341=CARTESIAN_POINT ( 'NONE',  ( 0.000000000000000000, 190.0000000000000000, 159.3522585083728700 ) ) ;
#28351=CARTESIAN_POINT ( 'NONE',  ( 0.000000000000000000, 190.0000000000000000, -2.000000000000000000 ) ) ;
#28367=DIRECTION ( 'NONE',  ( -0.000000000000000000, -0.000000000000000000, 1.000000000000000000 ) ) ;
#28389=VECTOR ( 'NONE', #55956, 1000.000000000000000 ) ;
#28403=VERTEX_POINT ( 'NONE', #64968 ) ;
#28428=LINE ( 'NONE', #2063, #35122 ) ;
#28432=VECTOR ( 'NONE', #59312, 1000.000000000000000 ) ;
#28456=CARTESIAN_POINT ( 'NONE',  ( 410.0000000000000000, 0.000000000000000000, -2.000000000000000000 ) ) ;
#28503=VERTEX_POINT ( 'NONE', #56142 ) ;
#28528=CARTESIAN_POINT ( 'NONE',  ( -17.50000000000002842, 207.5000000000000284, 0.000000000000000000 ) ) ;
#28546=VERTEX_POINT ( 'NONE', #34706 ) ;
#28548=ORIENTED_EDGE ( 'NONE', *, *, #33614, .F. ) ;
#28586=ORIENTED_EDGE ( 'NONE', *, *, #67836, .T. ) ;
#28650=LINE ( 'NONE', #39894, #22822 ) ;
#28668=VERTEX_POINT ( 'NONE', #35043 ) ;
#28683=AXIS2_PLACEMENT_3D ( 'NONE', #42280, #41587, #20822 ) ;
#28690=ORIENTED_EDGE ( 'NONE', *, *, #58213, .T. ) ;
#28694=AXIS2_PLACEMENT_3D ( 'NONE', #22044, #68837, #20661 ) ;
#28776=FACE_OUTER_BOUND ( 'NONE', #36380, .T. ) ;
#28781=ORIENTED_EDGE ( 'NONE', *, *, #23049, .T. ) ;
#28809=CARTESIAN_POINT ( 'NONE',  ( 154.4165763529819628, 225.8585178651493663, 138.9999999999999716 ) ) ;
#28814=CARTESIAN_POINT ( 'NONE',  ( 254.4165763529819344, 225.8585178651493948, 108.9999999999999858 ) ) ;
#28830=EDGE_LOOP ( 'NONE', ( #39796, #46515, #12708, #17147 ) ) ;
#28849=EDGE_CURVE ( 'NONE', #8603, #27646, #51739, .T. ) ;
#28865=EDGE_CURVE ( 'NONE', #9949, #40156, #61931, .T. ) ;
#28874=ORIENTED_EDGE ( 'NONE', *, *, #54778, .T. ) ;
#28920=LINE ( 'NONE', #45078, #12938 ) ;
#28956=AXIS2_PLACEMENT_3D ( 'NONE', #25602, #9757, #63221 ) ;
#28977=ORIENTED_EDGE ( 'NONE', *, *, #30021, .T. ) ;
#28989=EDGE_LOOP ( 'NONE', ( #12310, #35249, #21110, #9210, #60931, #43366 ) ) ;
#28990=ORIENTED_EDGE ( 'NONE', *, *, #67534, .T. ) ;
#29018=EDGE_CURVE ( 'NONE', #66152, #59483, #10841, .T. ) ;
#29022=DIRECTION ( 'NONE',  ( -0.000000000000000000, -0.000000000000000000, -1.000000000000000000 ) ) ;
#29037=CARTESIAN_POINT ( 'NONE',  ( 209.3223706822284100, 18.00000000000002842, 276.7520087653757628 ) ) ;
#29043=CARTESIAN_POINT ( 'NONE',  ( 307.2575771313985342, 172.0000000000000284, 256.6193948016162381 ) ) ;
#29074=DIRECTION ( 'NONE',  ( -0.000000000000000000, -0.9989683093773507050, -0.04541273895899305274 ) ) ;
#29089=LINE ( 'NONE', #44564, #15280 ) ;
#29108=CARTESIAN_POINT ( 'NONE',  ( 141.9165763529819344, -52.00000000000000711, 129.0000000000000000 ) ) ;
#29119=DIRECTION ( 'NONE',  ( -1.000000000000000000, 0.000000000000000000, 0.000000000000000000 ) ) ;
#29135=VECTOR ( 'NONE', #64554, 1000.000000000000000 ) ;
#29142=ORIENTED_EDGE ( 'NONE', *, *, #65773, .T. ) ;
#29159=ORIENTED_EDGE ( 'NONE', *, *, #35498, .F. ) ;
#29163=ORIENTED_EDGE ( 'NONE', *, *, #45999, .T. ) ;
#29187=DIRECTION ( 'NONE',  ( 0.000000000000000000, 0.000000000000000000, 1.000000000000000000 ) ) ;
#29188=CARTESIAN_POINT ( 'NONE',  ( 266.9165763529819628, 192.0000000000000000, 128.9999999999999716 ) ) ;
#29230=EDGE_CURVE ( 'NONE', #52338, #10473, #63936, .T. ) ;
#29247=DIRECTION ( 'NONE',  ( -0.000000000000000000, -0.000000000000000000, 1.000000000000000000 ) ) ;
#29259=CARTESIAN_POINT ( 'NONE',  ( -2.000000000000000000, 192.0000000000000000, 380.0000000000000000 ) ) ;
#29267=DIRECTION ( 'NONE',  ( -1.000000000000000000, 0.000000000000000000, 0.000000000000000000 ) ) ;
#29272=FACE_OUTER_BOUND ( 'NONE', #7088, .T. ) ;
#29286=CARTESIAN_POINT ( 'NONE',  ( 209.9999999999999716, -57.00000000000007816, 72.99999999999998579 ) ) ;
#29290=CARTESIAN_POINT ( 'NONE',  ( 149.4165763529819344, 225.8585178651493663, 129.0000000000000000 ) ) ;
#29292=CARTESIAN_POINT ( 'NONE',  ( 313.9975424824652350, 171.8183490441642789, 533.9018882243741473 ) ) ;
#29293=ORIENTED_EDGE ( 'NONE', *, *, #10854, .F. ) ;
#29315=FACE_OUTER_BOUND ( 'NONE', #54783, .T. ) ;
#29322=CARTESIAN_POINT ( 'NONE',  ( 111.9975424824652634, 172.0000000000000284, 418.0000000000000568 ) ) ;
#29373=ORIENTED_EDGE ( 'NONE', *, *, #314, .T. ) ;
#29374=CARTESIAN_POINT ( 'NONE',  ( 209.9999999999999716, -2.000000000000001776, 93.99999999999998579 ) ) ;
#29383=DIRECTION ( 'NONE',  ( 0.000000000000000000, -1.000000000000000000, 0.000000000000000000 ) ) ;
#29384=CYLINDRICAL_SURFACE ( 'NONE', #5289, 160.5210298272983778 ) ;
#29393=VERTEX_POINT ( 'NONE', #44195 ) ;
#29409=CIRCLE ( 'NONE', #68708, 5.000000000000000888 ) ;
#29416=CLOSED_SHELL ( 'NONE', ( #65442, #21674, #15577, #9048, #43735, #30186, #51291, #21931, #39105, #41389, #18142, #33465, #67887, #59542, #25438, #44372, #39551, #60362, #50185, #49449, #50491, #30197, #5221, #54619, #56902, #43553, #19046, #25817, #32780, #42317, #4321, #44384, #40582, #31534, #10074, #49605, #27093, #16267, #38973, #63611, #19806, #408, #51487, #59629, #32468, #13761, #22771, #31371, #62190, #59313, #21402, #64214, #26045, #19212, #31446, #41588, #50497, #48088, #43592, #63055, #48875, #51949, #66823, #39071, #68322, #21480, #20881, #25966, #57606, #289, #57978, #42480, #5090, #11126, #12707, #12472, #2105, #51064, #68297, #51711, #42999, #23672, #9938, #27489, #67823, #36617, #58134, #6598, #49849, #49454, #32320, #51762, #41543, #29623, #65471, #41687, #38701, #63551, #48314, #5634, #16882, #13739, #11319, #68778, #57864, #66091, #51071 ) ) ;
#29444=DIRECTION ( 'NONE',  ( -0.000000000000000000, 1.000000000000000000, -0.000000000000000000 ) ) ;
#29449=EDGE_CURVE ( 'NONE', #69450, #48350, #64628, .T. ) ;
#29507=ORIENTED_EDGE ( 'NONE', *, *, #13717, .T. ) ;
#29584=DIRECTION ( 'NONE',  ( -0.000000000000000000, -0.000000000000000000, -1.000000000000000000 ) ) ;
#29599=VERTEX_POINT ( 'NONE', #11067 ) ;
#29608=PLANE ( 'NONE',  #64024 ) ;
#29617=CARTESIAN_POINT ( 'NONE',  ( 311.9975424824652350, 296.0000000000000000, 529.9060149868646477 ) ) ;
#29623=ADVANCED_FACE ( 'NONE', ( #57284 ), #46364, .F. ) ;
#29665=CARTESIAN_POINT ( 'NONE',  ( 209.9999999999999716, 190.0000000000000000, 72.99999999999998579 ) ) ;
#29673=LINE ( 'NONE', #13501, #5334 ) ;
#29695=FACE_OUTER_BOUND ( 'NONE', #51167, .T. ) ;
#29699=AXIS2_PLACEMENT_3D ( 'NONE', #29932, #1822, #56312 ) ;
#29702=VECTOR ( 'NONE', #5038, 1000.000000000000000 ) ;
#29709=DIRECTION ( 'NONE',  ( -0.000000000000000000, -0.000000000000000000, 1.000000000000000000 ) ) ;
#29710=ORIENTED_EDGE ( 'NONE', *, *, #48395, .F. ) ;
#29711=DIRECTION ( 'NONE',  ( -1.000000000000000000, 0.000000000000000000, 0.000000000000000000 ) ) ;
#29725=VERTEX_POINT ( 'NONE', #23889 ) ;
#29729=CARTESIAN_POINT ( 'NONE',  ( 0.000000000000000000, 0.000000000000000000, -2.000000000000000000 ) ) ;
#29741=DIRECTION ( 'NONE',  ( 0.000000000000000000, 0.000000000000000000, 1.000000000000000000 ) ) ;
#29768=DIRECTION ( 'NONE',  ( 2.775557561562891844E-16, -0.000000000000000000, 1.000000000000000000 ) ) ;
#29809=CIRCLE ( 'NONE', #69098, 246.3582898394607241 ) ;
#29817=CARTESIAN_POINT ( 'NONE',  ( 141.9165763529819344, -2.000000000000001776, 129.0000000000000000 ) ) ;
#29844=CARTESIAN_POINT ( 'NONE',  ( 259.4165763529819060, -27.00000000000000355, 108.9999999999999858 ) ) ;
#29856=AXIS2_PLACEMENT_3D ( 'NONE', #43019, #42006, #11022 ) ;
#29863=EDGE_LOOP ( 'NONE', ( #46653, #49005, #33163, #63362, #10415, #66809, #56620, #27144 ) ) ;
#29869=ORIENTED_EDGE ( 'NONE', *, *, #9935, .T. ) ;
#29884=ORIENTED_EDGE ( 'NONE', *, *, #66713, .T. ) ;
#29886=ORIENTED_EDGE ( 'NONE', *, *, #473, .T. ) ;
#29895=VECTOR ( 'NONE', #61702, 1000.000000000000000 ) ;
#29900=VECTOR ( 'NONE', #38366, 1000.000000000000000 ) ;
#29913=CARTESIAN_POINT ( 'NONE',  ( -22.50000000000003197, -18.06806526123148160, 0.000000000000000000 ) ) ;
#29926=DIRECTION ( 'NONE',  ( -0.000000000000000000, -1.000000000000000000, -0.000000000000000000 ) ) ;
#29932=CARTESIAN_POINT ( 'NONE',  ( 149.4165763529819344, -26.99999999999998224, 138.9999999999999716 ) ) ;
#29967=FACE_OUTER_BOUND ( 'NONE', #51817, .T. ) ;
#30005=DIRECTION ( 'NONE',  ( -0.000000000000000000, 0.000000000000000000, 1.000000000000000000 ) ) ;
#30021=EDGE_CURVE ( 'NONE', #45190, #43728, #17111, .T. ) ;
#30059=CARTESIAN_POINT ( 'NONE',  ( 427.4999999999999432, 207.5000000000000284, 0.000000000000000000 ) ) ;
#30065=DIRECTION ( 'NONE',  ( -1.000000000000000000, 0.000000000000000000, 0.000000000000000000 ) ) ;
#30074=ORIENTED_EDGE ( 'NONE', *, *, #44302, .T. ) ;
#30090=VECTOR ( 'NONE', #16865, 1000.000000000000000 ) ;
#30092=DIRECTION ( 'NONE',  ( -0.000000000000000000, 0.000000000000000000, -1.000000000000000000 ) ) ;
#30100=CARTESIAN_POINT ( 'NONE',  ( 0.000000000000000000, 190.0000000000000000, 380.0000000000000000 ) ) ;
#30110=ORIENTED_EDGE ( 'NONE', *, *, #50417, .T. ) ;
#30165=ORIENTED_EDGE ( 'NONE', *, *, #28112, .F. ) ;
#30176=ORIENTED_EDGE ( 'NONE', *, *, #17201, .F. ) ;
#30186=ADVANCED_FACE ( 'NONE', ( #62028 ), #3989, .T. ) ;
#30197=ADVANCED_FACE ( 'NONE', ( #37031 ), #38059, .F. ) ;
#30240=CIRCLE ( 'NONE', #8903, 164.5210298272983778 ) ;
#30276=DIRECTION ( 'NONE',  ( 0.000000000000000000, 0.000000000000000000, -1.000000000000000000 ) ) ;
#30283=CARTESIAN_POINT ( 'NONE',  ( 313.9975424824652350, 18.00000000000002842, 256.6193948016162381 ) ) ;
#30294=CIRCLE ( 'NONE', #53854, 21.00000000000000355 ) ;
#30364=DIRECTION ( 'NONE',  ( 0.000000000000000000, 1.000000000000000000, -0.000000000000000000 ) ) ;
#30387=FACE_OUTER_BOUND ( 'NONE', #27352, .T. ) ;
#30393=CARTESIAN_POINT ( 'NONE',  ( 209.9999999999999716, 0.000000000000000000, 93.99999999999998579 ) ) ;
#30410=ORIENTED_EDGE ( 'NONE', *, *, #44466, .T. ) ;
#30478=CARTESIAN_POINT ( 'NONE',  ( -17.50000000000002842, -18.06806526123148160, -2.000000000000000000 ) ) ;
#30521=DIRECTION ( 'NONE',  ( 0.000000000000000000, 0.000000000000000000, -1.000000000000000000 ) ) ;
#30559=ORIENTED_EDGE ( 'NONE', *, *, #62279, .T. ) ;
#30572=CARTESIAN_POINT ( 'NONE',  ( 111.9975424824652634, 172.0000000000000284, 527.9060149868646477 ) ) ;
#30614=CARTESIAN_POINT ( 'NONE',  ( 230.9999999999999432, -35.00000000000000000, 0.000000000000000000 ) ) ;
#30637=LINE ( 'NONE', #20080, #41994 ) ;
#30661=FACE_OUTER_BOUND ( 'NONE', #1188, .T. ) ;
#30664=AXIS2_PLACEMENT_3D ( 'NONE', #43321, #64799, #44019 ) ;
#30668=VECTOR ( 'NONE', #6549, 1000.000000000000000 ) ;
#30672=DIRECTION ( 'NONE',  ( -0.000000000000000000, -0.000000000000000000, -1.000000000000000000 ) ) ;
#30673=ORIENTED_EDGE ( 'NONE', *, *, #5773, .T. ) ;
#30679=DIRECTION ( 'NONE',  ( -1.000000000000000000, 0.000000000000000000, 0.000000000000000000 ) ) ;
#30713=AXIS2_PLACEMENT_3D ( 'NONE', #33120, #6380, #27834 ) ;
#30754=DIRECTION ( 'NONE',  ( 0.000000000000000000, 0.000000000000000000, 1.000000000000000000 ) ) ;
#30762=VECTOR ( 'NONE', #14212, 1000.000000000000000 ) ;
#30784=EDGE_LOOP ( 'NONE', ( #63399, #25132 ) ) ;
#30805=VECTOR ( 'NONE', #33750, 1000.000000000000000 ) ;
#30821=LINE ( 'NONE', #52265, #58544 ) ;
#30840=EDGE_CURVE ( 'NONE', #54103, #7837, #57641, .T. ) ;
#30842=CARTESIAN_POINT ( 'NONE',  ( 109.9975424824652634, 18.00000000000002842, 536.6193948016162949 ) ) ;
#30856=CIRCLE ( 'NONE', #32005, 5.000000000000000888 ) ;
#30902=EDGE_CURVE ( 'NONE', #36681, #14130, #27684, .T. ) ;
#30930=VERTEX_POINT ( 'NONE', #56163 ) ;
#30973=DIRECTION ( 'NONE',  ( 1.000000000000000000, -0.000000000000000000, -0.000000000000000000 ) ) ;
#30986=LINE ( 'NONE', #21443, #16176 ) ;
#30989=EDGE_CURVE ( 'NONE', #8357, #2382, #24168, .T. ) ;
#30991=VERTEX_POINT ( 'NONE', #45955 ) ;
#31061=DIRECTION ( 'NONE',  ( -0.000000000000000000, -0.000000000000000000, -1.000000000000000000 ) ) ;
#31078=DIRECTION ( 'NONE',  ( 1.000000000000000000, 0.000000000000000000, -0.000000000000000000 ) ) ;
#31105=FACE_BOUND ( 'NONE', #52074, .T. ) ;
#31148=DIRECTION ( 'NONE',  ( -0.000000000000000000, -0.000000000000000000, -1.000000000000000000 ) ) ;
#31211=VECTOR ( 'NONE', #64068, 1000.000000000000000 ) ;
#31230=ORIENTED_EDGE ( 'NONE', *, *, #45253, .F. ) ;
#31241=VERTEX_POINT ( 'NONE', #65242 ) ;
#31254=AXIS2_PLACEMENT_3D ( 'NONE', #345, #37990, #16536 ) ;
#31269=LINE ( 'NONE', #15079, #64867 ) ;
#31292=CARTESIAN_POINT ( 'NONE',  ( 109.9975424824652777, 296.0000000000000000, 418.0000000000000000 ) ) ;
#31297=ORIENTED_EDGE ( 'NONE', *, *, #64162, .T. ) ;
#31332=ORIENTED_EDGE ( 'NONE', *, *, #53903, .F. ) ;
#31371=ADVANCED_FACE ( 'NONE', ( #29695 ), #51161, .F. ) ;
#31388=ORIENTED_EDGE ( 'NONE', *, *, #15301, .F. ) ;
#31411=DIRECTION ( 'NONE',  ( -0.000000000000000000, 1.000000000000000000, -0.000000000000000000 ) ) ;
#31413=CARTESIAN_POINT ( 'NONE',  ( 230.9999999999999432, -57.00000000000007816, -2.000000000000000000 ) ) ;
#31423=DIRECTION ( 'NONE',  ( -0.000000000000000000, -0.000000000000000000, -1.000000000000000000 ) ) ;
#31446=ADVANCED_FACE ( 'NONE', ( #55377 ), #52187, .F. ) ;
#31447=ORIENTED_EDGE ( 'NONE', *, *, #45675, .F. ) ;
#31474=CIRCLE ( 'NONE', #53891, 5.000000000000004441 ) ;
#31482=VERTEX_POINT ( 'NONE', #59432 ) ;
#31483=CARTESIAN_POINT ( 'NONE',  ( 109.9975424824652634, 295.6904194069557548, 539.5330678552892323 ) ) ;
#31511=VERTEX_POINT ( 'NONE', #62401 ) ;
#31527=LINE ( 'NONE', #53988, #58907 ) ;
#31534=ADVANCED_FACE ( 'NONE', ( #57467, #8940, #25473, #3653, #53800, #30387 ), #25126, .T. ) ;
#31551=FACE_OUTER_BOUND ( 'NONE', #25323, .T. ) ;
#31656=EDGE_LOOP ( 'NONE', ( #38987, #15750 ) ) ;
#31714=DIRECTION ( 'NONE',  ( -0.000000000000000000, -0.000000000000000000, -1.000000000000000000 ) ) ;
#31722=ORIENTED_EDGE ( 'NONE', *, *, #64162, .F. ) ;
#31749=VECTOR ( 'NONE', #61143, 1000.000000000000000 ) ;
#31775=LINE ( 'NONE', #53208, #29702 ) ;
#31778=ORIENTED_EDGE ( 'NONE', *, *, #67836, .F. ) ;
#31787=EDGE_CURVE ( 'NONE', #14720, #67398, #51677, .T. ) ;
#31791=CARTESIAN_POINT ( 'NONE',  ( -17.50000000000002842, -18.06806526123148160, 378.0000000000000000 ) ) ;
#31808=CARTESIAN_POINT ( 'NONE',  ( -17.50000000000002842, 207.5000000000000284, 380.0000000000000000 ) ) ;
#31824=ORIENTED_EDGE ( 'NONE', *, *, #39110, .T. ) ;
#31831=ORIENTED_EDGE ( 'NONE', *, *, #55743, .T. ) ;
#31854=AXIS2_PLACEMENT_3D ( 'NONE', #44971, #60459, #50597 ) ;
#31862=CARTESIAN_POINT ( 'NONE',  ( -2.000000000000000000, 192.0000000000000000, 378.0000000000000000 ) ) ;
#31865=DIRECTION ( 'NONE',  ( -1.000000000000000000, 0.000000000000000000, 2.220446049250313081E-16 ) ) ;
#31922=VECTOR ( 'NONE', #31411, 1000.000000000000000 ) ;
#31931=EDGE_CURVE ( 'NONE', #69411, #38117, #42824, .T. ) ;
#31954=CARTESIAN_POINT ( 'NONE',  ( 311.9975424824652350, 22.00669820036272384, 401.6295345748407613 ) ) ;
#31966=ORIENTED_EDGE ( 'NONE', *, *, #68240, .F. ) ;
#31972=CARTESIAN_POINT ( 'NONE',  ( 111.9975424824652634, 170.0000000000000284, 354.1673509436691347 ) ) ;
#31975=ORIENTED_EDGE ( 'NONE', *, *, #3843, .F. ) ;
#31980=EDGE_CURVE ( 'NONE', #1198, #40354, #65699, .T. ) ;
#32003=AXIS2_PLACEMENT_3D ( 'NONE', #15460, #52055, #62952 ) ;
#32005=AXIS2_PLACEMENT_3D ( 'NONE', #48944, #37717, #10983 ) ;
#32026=DIRECTION ( 'NONE',  ( 1.000000000000000000, 0.000000000000000000, -0.000000000000000000 ) ) ;
#32040=ORIENTED_EDGE ( 'NONE', *, *, #51706, .F. ) ;
#32054=CARTESIAN_POINT ( 'NONE',  ( 259.4165763529819060, 225.8585178651493948, 128.9999999999999716 ) ) ;
#32089=CARTESIAN_POINT ( 'NONE',  ( 209.9518228411288874, 190.0000000000000000, 31.43423095485942298 ) ) ;
#32094=EDGE_CURVE ( 'NONE', #67398, #47824, #12228, .T. ) ;
#32118=ORIENTED_EDGE ( 'NONE', *, *, #64631, .T. ) ;
#32145=VECTOR ( 'NONE', #50546, 1000.000000000000000 ) ;
#32182=CARTESIAN_POINT ( 'NONE',  ( 230.9999999999999432, 225.0000000000000000, 0.000000000000000000 ) ) ;
#32195=CIRCLE ( 'NONE', #16467, 246.3582898394606957 ) ;
#32229=ORIENTED_EDGE ( 'NONE', *, *, #35498, .T. ) ;
#32243=VERTEX_POINT ( 'NONE', #31862 ) ;
#32249=CARTESIAN_POINT ( 'NONE',  ( 444.9999999999999432, 225.0000000000000000, 0.000000000000000000 ) ) ;
#32291=VECTOR ( 'NONE', #45002, 1000.000000000000114 ) ;
#32299=CARTESIAN_POINT ( 'NONE',  ( 311.9975424824652350, 170.0000000000000284, 255.6641978984094408 ) ) ;
#32302=FACE_OUTER_BOUND ( 'NONE', #33730, .T. ) ;
#32306=LINE ( 'NONE', #17500, #18270 ) ;
#32320=ADVANCED_FACE ( 'NONE', ( #27612 ), #54692, .T. ) ;
#32368=LINE ( 'NONE', #42570, #30090 ) ;
#32393=EDGE_CURVE ( 'NONE', #61540, #61512, #60326, .T. ) ;
#32406=DIRECTION ( 'NONE',  ( 0.000000000000000000, 0.000000000000000000, 1.000000000000000000 ) ) ;
#32462=FACE_OUTER_BOUND ( 'NONE', #8279, .T. ) ;
#32465=ORIENTED_EDGE ( 'NONE', *, *, #52861, .F. ) ;
#32468=ADVANCED_FACE ( 'NONE', ( #59269 ), #5805, .F. ) ;
#32481=EDGE_CURVE ( 'NONE', #42236, #9171, #7911, .T. ) ;
#32548=DIRECTION ( 'NONE',  ( 0.000000000000000000, -0.04541273895899431562, 0.9989683093773507050 ) ) ;
#32572=EDGE_CURVE ( 'NONE', #41662, #45190, #2986, .T. ) ;
#32589=CARTESIAN_POINT ( 'NONE',  ( 266.9165763529819628, -2.000000000000001776, 128.9999999999999716 ) ) ;
#32600=CARTESIAN_POINT ( 'NONE',  ( 410.0000000000000000, 0.000000000000000000, 175.2157797990580832 ) ) ;
#32656=EDGE_LOOP ( 'NONE', ( #53943, #66107, #17669, #28021 ) ) ;
#32668=CARTESIAN_POINT ( 'NONE',  ( 209.9999999999999716, 190.0000000000000000, 72.99999999999998579 ) ) ;
#32727=ORIENTED_EDGE ( 'NONE', *, *, #7254, .T. ) ;
#32729=VERTEX_POINT ( 'NONE', #53210 ) ;
#32731=ORIENTED_EDGE ( 'NONE', *, *, #39463, .T. ) ;
#32744=PLANE ( 'NONE',  #13633 ) ;
#32780=ADVANCED_FACE ( 'NONE', ( #64128 ), #19848, .T. ) ;
#32822=CARTESIAN_POINT ( 'NONE',  ( -35.00000000000002842, -35.00000000000000000, -2.000000000000000000 ) ) ;
#32826=CYLINDRICAL_SURFACE ( 'NONE', #6679, 5.000000000000000888 ) ;
#32846=CARTESIAN_POINT ( 'NONE',  ( -17.50000000000002842, 207.5000000000000284, 378.0000000000000000 ) ) ;
#32866=VECTOR ( 'NONE', #19945, 1000.000000000000000 ) ;
#32870=CARTESIAN_POINT ( 'NONE',  ( -35.00000000000002842, -35.00000000000000000, 378.0000000000000000 ) ) ;
#32892=EDGE_LOOP ( 'NONE', ( #10007, #58609, #38077, #16098 ) ) ;
#32899=VECTOR ( 'NONE', #4993, 1000.000000000000114 ) ;
#32916=EDGE_CURVE ( 'NONE', #25612, #31482, #67283, .T. ) ;
#32919=DIRECTION ( 'NONE',  ( 0.000000000000000000, 0.02271222823333338484, -0.9997420440737084801 ) ) ;
#32939=EDGE_LOOP ( 'NONE', ( #33949, #65244, #13452, #19383, #11432, #23553, #65026, #41816, #23541, #9322, #23354, #684 ) ) ;
#32988=FACE_OUTER_BOUND ( 'NONE', #48887, .T. ) ;
#32993=LINE ( 'NONE', #54430, #54024 ) ;
#33004=AXIS2_PLACEMENT_3D ( 'NONE', #34702, #17454, #66374 ) ;
#33019=DIRECTION ( 'NONE',  ( -0.000000000000000000, -0.000000000000000000, -1.000000000000000000 ) ) ;
#33025=ORIENTED_EDGE ( 'NONE', *, *, #24226, .F. ) ;
#33046=DIRECTION ( 'NONE',  ( 1.000000000000000000, 0.000000000000000000, 0.000000000000000000 ) ) ;
#33051=EDGE_CURVE ( 'NONE', #46092, #28503, #52295, .T. ) ;
#33064=DIRECTION ( 'NONE',  ( -1.000000000000000000, 0.000000000000000000, 0.000000000000000000 ) ) ;
#33065=AXIS2_PLACEMENT_3D ( 'NONE', #63758, #64091, #15566 ) ;
#33084=CARTESIAN_POINT ( 'NONE',  ( 422.4999999999999432, -18.06806526123148160, 378.0000000000000000 ) ) ;
#33088=FACE_OUTER_BOUND ( 'NONE', #68951, .T. ) ;
#33120=CARTESIAN_POINT ( 'NONE',  ( 209.3223706822284100, 190.0000000000000000, 31.44247402469554942 ) ) ;
#33163=ORIENTED_EDGE ( 'NONE', *, *, #39086, .T. ) ;
#33196=EDGE_CURVE ( 'NONE', #13211, #7345, #30240, .T. ) ;
#33200=CARTESIAN_POINT ( 'NONE',  ( 410.0000000000000000, 0.000000000000000000, 380.0000000000000000 ) ) ;
#33212=LINE ( 'NONE', #55344, #55444 ) ;
#33216=LINE ( 'NONE', #39191, #56176 ) ;
#33254=CIRCLE ( 'NONE', #52375, 5.000000000000004441 ) ;
#33270=EDGE_CURVE ( 'NONE', #69128, #24965, #22356, .T. ) ;
#33291=CARTESIAN_POINT ( 'NONE',  ( 311.9975424824652350, 170.0000000000000284, 380.0000000000001137 ) ) ;
#33294=VERTEX_POINT ( 'NONE', #38896 ) ;
#33298=DIRECTION ( 'NONE',  ( -0.000000000000000000, -1.000000000000000000, 0.000000000000000000 ) ) ;
#33299=DIRECTION ( 'NONE',  ( 0.000000000000000000, 1.000000000000000000, 0.000000000000000000 ) ) ;
#33344=ORIENTED_EDGE ( 'NONE', *, *, #68283, .F. ) ;
#33368=VERTEX_POINT ( 'NONE', #29043 ) ;
#33403=ORIENTED_EDGE ( 'NONE', *, *, #37677, .T. ) ;
#33449=CIRCLE ( 'NONE', #51426, 5.000000000000004441 ) ;
#33465=ADVANCED_FACE ( 'NONE', ( #54618 ), #32826, .F. ) ;
#33504=FACE_OUTER_BOUND ( 'NONE', #15986, .T. ) ;
#33509=AXIS2_PLACEMENT_3D ( 'NONE', #31413, #31078, #9616 ) ;
#33515=LINE ( 'NONE', #6761, #38630 ) ;
#33523=DIRECTION ( 'NONE',  ( -1.000000000000000000, 0.000000000000000000, 0.000000000000000000 ) ) ;
#33536=PLANE ( 'NONE',  #68704 ) ;
#33562=CARTESIAN_POINT ( 'NONE',  ( 109.9975424824652634, 295.6904194069557548, 539.5330678552892323 ) ) ;
#33565=AXIS2_PLACEMENT_3D ( 'NONE', #44127, #6151, #32548 ) ;
#33581=CARTESIAN_POINT ( 'NONE',  ( 259.4165763529819060, -27.00000000000000355, 138.9999999999999716 ) ) ;
#33607=DIRECTION ( 'NONE',  ( 0.000000000000000000, 0.000000000000000000, 1.000000000000000000 ) ) ;
#33613=VECTOR ( 'NONE', #19147, 1000.000000000000000 ) ;
#33614=EDGE_CURVE ( 'NONE', #62679, #46362, #30294, .T. ) ;
#33633=EDGE_CURVE ( 'NONE', #62233, #37433, #48981, .T. ) ;
#33656=ORIENTED_EDGE ( 'NONE', *, *, #64022, .T. ) ;
#33702=LINE ( 'NONE', #44225, #35086 ) ;
#33708=EDGE_LOOP ( 'NONE', ( #37221, #10559, #22264, #4797 ) ) ;
#33730=EDGE_LOOP ( 'NONE', ( #69044, #61629, #55979, #9881, #59599, #26907, #13597, #65941, #23383, #10402, #50581, #53161 ) ) ;
#33738=DIRECTION ( 'NONE',  ( -0.000000000000000000, -0.000000000000000000, 1.000000000000000000 ) ) ;
#33745=DIRECTION ( 'NONE',  ( 0.000000000000000000, -1.000000000000000000, 0.000000000000000000 ) ) ;
#33750=DIRECTION ( 'NONE',  ( -0.000000000000000000, -1.000000000000000000, 0.000000000000000000 ) ) ;
#33768=EDGE_CURVE ( 'NONE', #17316, #2210, #3945, .T. ) ;
#33788=DIRECTION ( 'NONE',  ( 1.000000000000000000, 0.000000000000000000, 0.000000000000000000 ) ) ;
#33812=ORIENTED_EDGE ( 'NONE', *, *, #46043, .T. ) ;
#33831=AXIS2_PLACEMENT_3D ( 'NONE', #54621, #11360, #22622 ) ;
#33838=EDGE_LOOP ( 'NONE', ( #8654, #27814 ) ) ;
#33849=DIRECTION ( 'NONE',  ( -0.000000000000000000, -0.000000000000000000, -1.000000000000000000 ) ) ;
#33886=ORIENTED_EDGE ( 'NONE', *, *, #27631, .T. ) ;
#33921=VECTOR ( 'NONE', #45436, 1000.000000000000000 ) ;
#33930=CYLINDRICAL_SURFACE ( 'NONE', #10491, 21.00000000000000355 ) ;
#33949=ORIENTED_EDGE ( 'NONE', *, *, #10636, .F. ) ;
#33974=LINE ( 'NONE', #66693, #18638 ) ;
#34004=EDGE_CURVE ( 'NONE', #17967, #47060, #14537, .T. ) ;
#34027=VECTOR ( 'NONE', #15374, 1000.000000000000000 ) ;
#34034=DIRECTION ( 'NONE',  ( -0.000000000000000000, -0.000000000000000000, -1.000000000000000000 ) ) ;
#34049=ORIENTED_EDGE ( 'NONE', *, *, #12471, .F. ) ;
#34083=AXIS2_PLACEMENT_3D ( 'NONE', #47152, #48512, #32026 ) ;
#34094=DIRECTION ( 'NONE',  ( 0.000000000000000000, -1.000000000000000000, 0.000000000000000000 ) ) ;
#34096=DIRECTION ( 'NONE',  ( -0.000000000000000000, -1.000000000000000000, -0.000000000000000000 ) ) ;
#34110=LINE ( 'NONE', #1750, #39073 ) ;
#34120=ORIENTED_EDGE ( 'NONE', *, *, #11262, .T. ) ;
#34129=AXIS2_PLACEMENT_3D ( 'NONE', #37251, #58702, #53767 ) ;
#34136=AXIS2_PLACEMENT_3D ( 'NONE', #49217, #22503, #33064 ) ;
#34178=CARTESIAN_POINT ( 'NONE',  ( 432.4999999999999432, -18.06806526123148160, 380.0000000000000000 ) ) ;
#34200=DIRECTION ( 'NONE',  ( -0.000000000000000000, -0.9989683093773507050, -0.04541273895899305274 ) ) ;
#34236=FACE_OUTER_BOUND ( 'NONE', #37786, .T. ) ;
#34271=DIRECTION ( 'NONE',  ( -1.000000000000000000, 0.000000000000000000, 0.000000000000000000 ) ) ;
#34313=VERTEX_POINT ( 'NONE', #7329 ) ;
#34316=CIRCLE ( 'NONE', #43261, 245.3095347406802205 ) ;
#34320=CIRCLE ( 'NONE', #3987, 246.3582898394607525 ) ;
#34328=PLANE ( 'NONE',  #10996 ) ;
#34335=CARTESIAN_POINT ( 'NONE',  ( 311.9975424824652350, 172.0000000000000284, 418.0000000000000568 ) ) ;
#34359=LINE ( 'NONE', #6566, #35224 ) ;
#34367=ORIENTED_EDGE ( 'NONE', *, *, #12858, .T. ) ;
#34368=LINE ( 'NONE', #44905, #42984 ) ;
#34376=EDGE_LOOP ( 'NONE', ( #28690, #58528, #4717, #17806, #29869, #58844, #17165, #4716 ) ) ;
#34394=VERTEX_POINT ( 'NONE', #36134 ) ;
#34395=DIRECTION ( 'NONE',  ( -0.000000000000000000, -0.000000000000000000, -1.000000000000000000 ) ) ;
#34472=PRODUCT ( 'Part1', 'Part1', '', ( #43074 ) ) ;
#34485=ORIENTED_EDGE ( 'NONE', *, *, #59443, .F. ) ;
#34487=EDGE_CURVE ( 'NONE', #5133, #55571, #52980, .T. ) ;
#34539=EDGE_LOOP ( 'NONE', ( #62675, #57214, #4573, #24456 ) ) ;
#34562=DIRECTION ( 'NONE',  ( -1.000000000000000000, 0.000000000000000000, 0.000000000000000000 ) ) ;
#34702=CARTESIAN_POINT ( 'NONE',  ( 309.8720357909272707, 172.0000000000000284, 536.6193948016162949 ) ) ;
#34706=CARTESIAN_POINT ( 'NONE',  ( 412.0000000000000000, 192.0000000000000000, 378.0000000000000000 ) ) ;
#34756=VERTEX_POINT ( 'NONE', #20816 ) ;
#34768=CARTESIAN_POINT ( 'NONE',  ( 111.9975424824652634, 295.8720703627916464, 535.5371946177799600 ) ) ;
#34791=ORIENTED_EDGE ( 'NONE', *, *, #69395, .T. ) ;
#34816=ORIENTED_EDGE ( 'NONE', *, *, #61409, .F. ) ;
#34851=ORIENTED_EDGE ( 'NONE', *, *, #39110, .F. ) ;
#34853=LINE ( 'NONE', #39087, #28389 ) ;
#34918=ORIENTED_EDGE ( 'NONE', *, *, #7336, .F. ) ;
#34922=DIRECTION ( 'NONE',  ( -0.9216045519012663334, 0.000000000000000000, 0.3881301971180111110 ) ) ;
#34950=CARTESIAN_POINT ( 'NONE',  ( 141.9165763529819344, 192.0000000000000000, 129.0000000000000000 ) ) ;
#34964=ORIENTED_EDGE ( 'NONE', *, *, #48079, .T. ) ;
#34988=ORIENTED_EDGE ( 'NONE', *, *, #40030, .F. ) ;
#35011=FACE_BOUND ( 'NONE', #230, .T. ) ;
#35043=CARTESIAN_POINT ( 'NONE',  ( 211.9975424824652066, 190.0000000000000284, 276.7368757365948682 ) ) ;
#35064=DIRECTION ( 'NONE',  ( 0.000000000000000000, 0.000000000000000000, -1.000000000000000000 ) ) ;
#35075=LINE ( 'NONE', #13286, #63442 ) ;
#35079=EDGE_LOOP ( 'NONE', ( #41070, #50547, #46010, #12357 ) ) ;
#35086=VECTOR ( 'NONE', #43182, 1000.000000000000000 ) ;
#35099=CARTESIAN_POINT ( 'NONE',  ( 209.9518228411288874, 0.000000000000000000, 31.43423095485942298 ) ) ;
#35122=VECTOR ( 'NONE', #61491, 1000.000000000000114 ) ;
#35171=EDGE_CURVE ( 'NONE', #25214, #20810, #42194, .T. ) ;
#35195=VERTEX_POINT ( 'NONE', #18579 ) ;
#35203=LINE ( 'NONE', #52744, #38988 ) ;
#35213=DIRECTION ( 'NONE',  ( -0.000000000000000000, -0.000000000000000000, 1.000000000000000000 ) ) ;
#35224=VECTOR ( 'NONE', #28012, 1000.000000000000000 ) ;
#35249=ORIENTED_EDGE ( 'NONE', *, *, #30902, .T. ) ;
#35253=EDGE_LOOP ( 'NONE', ( #21425, #9214, #68577, #55084, #57918, #8434, #34988, #65062, #42741, #59159, #4438, #27066 ) ) ;
#35264=DIRECTION ( 'NONE',  ( 1.000000000000000000, 0.000000000000000000, -2.220446049250313081E-16 ) ) ;
#35266=AXIS2_PLACEMENT_3D ( 'NONE', #20842, #25101, #4333 ) ;
#35311=DIRECTION ( 'NONE',  ( -0.000000000000000000, -0.000000000000000000, 1.000000000000000000 ) ) ;
#35341=LINE ( 'NONE', #56800, #606 ) ;
#35394=DIRECTION ( 'NONE',  ( 0.000000000000000000, 0.000000000000000000, 1.000000000000000000 ) ) ;
#35422=AXIS2_PLACEMENT_3D ( 'NONE', #17288, #49638, #65851 ) ;
#35468=DIRECTION ( 'NONE',  ( -0.000000000000000000, 1.000000000000000000, -0.000000000000000000 ) ) ;
#35474=ORIENTED_EDGE ( 'NONE', *, *, #23599, .F. ) ;
#35480=EDGE_LOOP ( 'NONE', ( #32727, #12807, #20507, #23481, #34049, #62747, #35708, #51964 ) ) ;
#35498=EDGE_CURVE ( 'NONE', #69361, #43260, #14633, .T. ) ;
#35501=ORIENTED_EDGE ( 'NONE', *, *, #67054, .T. ) ;
#35534=LINE ( 'NONE', #4549, #56318 ) ;
#35579=EDGE_CURVE ( 'NONE', #14950, #46092, #45594, .T. ) ;
#35584=PLANE ( 'NONE',  #6421 ) ;
#35594=EDGE_LOOP ( 'NONE', ( #24631, #47708, #5815, #31831 ) ) ;
#35595=DIRECTION ( 'NONE',  ( 0.000000000000000000, -0.000000000000000000, 1.000000000000000000 ) ) ;
#35609=VERTEX_POINT ( 'NONE', #51558 ) ;
#35617=VECTOR ( 'NONE', #60395, 1000.000000000000000 ) ;
#35637=ORIENTED_EDGE ( 'NONE', *, *, #3263, .F. ) ;
#35641=DIRECTION ( 'NONE',  ( 0.000000000000000000, -0.9940777367219241212, 0.1086713087885527174 ) ) ;
#35648=PLANE ( 'NONE',  #61043 ) ;
#35708=ORIENTED_EDGE ( 'NONE', *, *, #11809, .T. ) ;
#35763=ORIENTED_EDGE ( 'NONE', *, *, #14979, .T. ) ;
#35782=ORIENTED_EDGE ( 'NONE', *, *, #67937, .F. ) ;
#35823=CARTESIAN_POINT ( 'NONE',  ( 209.9999999999999716, -2.000000000000001776, 72.99999999999998579 ) ) ;
#35830=DIRECTION ( 'NONE',  ( 2.220446049250313081E-16, -0.000000000000000000, 1.000000000000000000 ) ) ;
#35904=VERTEX_POINT ( 'NONE', #50081 ) ;
#35927=CARTESIAN_POINT ( 'NONE',  ( 410.0000000000000000, 0.000000000000000000, 380.0000000000000000 ) ) ;
#35939=ORIENTED_EDGE ( 'NONE', *, *, #58675, .F. ) ;
#36009=CARTESIAN_POINT ( 'NONE',  ( 444.9999999999999432, 225.0000000000000000, 378.0000000000000000 ) ) ;
#36018=ORIENTED_EDGE ( 'NONE', *, *, #15097, .F. ) ;
#36024=CYLINDRICAL_SURFACE ( 'NONE', #14736, 5.000000000000004441 ) ;
#36046=VECTOR ( 'NONE', #46274, 1000.000000000000227 ) ;
#36064=EDGE_CURVE ( 'NONE', #36681, #69450, #62987, .T. ) ;
#36065=CYLINDRICAL_SURFACE ( 'NONE', #2641, 5.000000000000004441 ) ;
#36074=LINE ( 'NONE', #12023, #42190 ) ;
#36110=ORIENTED_EDGE ( 'NONE', *, *, #20168, .T. ) ;
#36125=ORIENTED_EDGE ( 'NONE', *, *, #37793, .F. ) ;
#36134=CARTESIAN_POINT ( 'NONE',  ( 111.9975424824652634, 172.0000000000000284, 354.1673509436691347 ) ) ;
#36154=DIRECTION ( 'NONE',  ( -0.8496664383351307803, 0.000000000000000000, 0.5273205320930463014 ) ) ;
#36155=CARTESIAN_POINT ( 'NONE',  ( 444.9999999999999432, -35.00000000000000000, 378.0000000000000000 ) ) ;
#36159=LINE ( 'NONE', #57618, #112 ) ;
#36176=EDGE_LOOP ( 'NONE', ( #155, #22600, #46941, #2674 ) ) ;
#36238=LINE ( 'NONE', #62631, #22921 ) ;
#36277=ORIENTED_EDGE ( 'NONE', *, *, #29018, .T. ) ;
#36303=DIRECTION ( 'NONE',  ( -1.000000000000000000, 0.000000000000000000, -0.000000000000000000 ) ) ;
#36317=VERTEX_POINT ( 'NONE', #2008 ) ;
#36335=ORIENTED_EDGE ( 'NONE', *, *, #29449, .T. ) ;
#36340=VECTOR ( 'NONE', #56211, 1000.000000000000000 ) ;
#36363=EDGE_LOOP ( 'NONE', ( #42052, #20923 ) ) ;
#36364=EDGE_LOOP ( 'NONE', ( #2727, #21488, #23666, #39275, #10486, #25386, #63825, #48843 ) ) ;
#36370=FACE_BOUND ( 'NONE', #26549, .T. ) ;
#36373=EDGE_CURVE ( 'NONE', #13843, #38713, #45593, .T. ) ;
#36380=EDGE_LOOP ( 'NONE', ( #59331, #31966, #65287, #51031, #56096, #39901, #59232, #47612, #42703, #46348 ) ) ;
#36462=EDGE_LOOP ( 'NONE', ( #37598, #12635, #25807, #22195 ) ) ;
#36497=VERTEX_POINT ( 'NONE', #26558 ) ;
#36576=AXIS2_PLACEMENT_3D ( 'NONE', #32089, #26811, #39447 ) ;
#36587=CARTESIAN_POINT ( 'NONE',  ( 109.9975424824652634, 179.2896996249788799, 369.5505932007772003 ) ) ;
#36617=ADVANCED_FACE ( 'NONE', ( #38408 ), #10629, .T. ) ;
#36630=ORIENTED_EDGE ( 'NONE', *, *, #18444, .T. ) ;
#36648=DIRECTION ( 'NONE',  ( 1.000000000000000000, 0.000000000000000000, 0.000000000000000000 ) ) ;
#36652=ORIENTED_EDGE ( 'NONE', *, *, #51091, .F. ) ;
#36669=DIRECTION ( 'NONE',  ( -1.000000000000000000, 0.000000000000000000, 0.000000000000000000 ) ) ;
#36681=VERTEX_POINT ( 'NONE', #18177 ) ;
#36712=ORIENTED_EDGE ( 'NONE', *, *, #54467, .T. ) ;
#36717=EDGE_LOOP ( 'NONE', ( #36652, #49339, #39067, #7665 ) ) ;
#36751=EDGE_LOOP ( 'NONE', ( #6232, #65676, #26456, #4894 ) ) ;
#36783=DIRECTION ( 'NONE',  ( 0.000000000000000000, 0.000000000000000000, -1.000000000000000000 ) ) ;
#36802=FACE_BOUND ( 'NONE', #15488, .T. ) ;
#36818=VECTOR ( 'NONE', #54759, 1000.000000000000000 ) ;
#36827=CIRCLE ( 'NONE', #22211, 5.000000000000004441 ) ;
#36844=LINE ( 'NONE', #58283, #8578 ) ;
#36869=AXIS2_PLACEMENT_3D ( 'NONE', #20178, #4006, #19837 ) ;
#36902=ORIENTED_EDGE ( 'NONE', *, *, #35171, .F. ) ;
#36911=ORIENTED_EDGE ( 'NONE', *, *, #12412, .F. ) ;
#36949=EDGE_CURVE ( 'NONE', #5435, #18335, #50287, .T. ) ;
#36971=AXIS2_PLACEMENT_3D ( 'NONE', #2751, #49522, #1357 ) ;
#36972=EDGE_LOOP ( 'NONE', ( #12390, #36335, #41328, #16054 ) ) ;
#36990=CARTESIAN_POINT ( 'NONE',  ( 209.9518228411288874, 20.00000000000003197, 31.43423095485942298 ) ) ;
#37016=CARTESIAN_POINT ( 'NONE',  ( 311.9975424824652350, 20.00000000000003197, 380.0000000000001137 ) ) ;
#37031=FACE_OUTER_BOUND ( 'NONE', #49230, .T. ) ;
#37038=EDGE_CURVE ( 'NONE', #44856, #38713, #30821, .T. ) ;
#37041=DIRECTION ( 'NONE',  ( 0.000000000000000000, 0.000000000000000000, 1.000000000000000000 ) ) ;
#37046=AXIS2_PLACEMENT_3D ( 'NONE', #6634, #42862, #10865 ) ;
#37091=CARTESIAN_POINT ( 'NONE',  ( 141.9165763529819344, -52.00000000000000711, 129.0000000000000000 ) ) ;
#37092=CIRCLE ( 'NONE', #6764, 5.000000000000004441 ) ;
#37152=EDGE_CURVE ( 'NONE', #8163, #26255, #46205, .T. ) ;
#37164=VECTOR ( 'NONE', #7965, 1000.000000000000000 ) ;
#37182=PLANE ( 'NONE',  #28694 ) ;
#37221=ORIENTED_EDGE ( 'NONE', *, *, #27376, .T. ) ;
#37250=ORIENTED_EDGE ( 'NONE', *, *, #67937, .T. ) ;
#37251=CARTESIAN_POINT ( 'NONE',  ( -17.50000000000002842, 207.5000000000000284, 378.0000000000000000 ) ) ;
#37267=LINE ( 'NONE', #54124, #617 ) ;
#37318=PLANE ( 'NONE',  #2947 ) ;
#37321=EDGE_CURVE ( 'NONE', #35904, #18015, #8005, .T. ) ;
#37354=AXIS2_PLACEMENT_3D ( 'NONE', #11088, #65888, #31865 ) ;
#37360=CIRCLE ( 'NONE', #51941, 21.00000000000000355 ) ;
#37368=EDGE_CURVE ( 'NONE', #27491, #5170, #24768, .T. ) ;
#37382=LINE ( 'NONE', #10652, #49561 ) ;
#37385=VERTEX_POINT ( 'NONE', #62397 ) ;
#37404=FACE_OUTER_BOUND ( 'NONE', #7832, .T. ) ;
#37413=DIRECTION ( 'NONE',  ( -1.000000000000000000, 0.000000000000000000, 0.000000000000000000 ) ) ;
#37433=VERTEX_POINT ( 'NONE', #41628 ) ;
#37434=ORIENTED_EDGE ( 'NONE', *, *, #67514, .F. ) ;
#37453=CIRCLE ( 'NONE', #4875, 21.00000000000000355 ) ;
#37470=VECTOR ( 'NONE', #48779, 1000.000000000000000 ) ;
#37473=VERTEX_POINT ( 'NONE', #36009 ) ;
#37478=CARTESIAN_POINT ( 'NONE',  ( 0.000000000000000000, -2.000000000000000000, -0.000000000000000000 ) ) ;
#37497=EDGE_CURVE ( 'NONE', #40354, #5206, #12579, .T. ) ;
#37512=DIRECTION ( 'NONE',  ( -1.000000000000000000, 0.000000000000000000, 0.000000000000000000 ) ) ;
#37572=CIRCLE ( 'NONE', #60115, 245.3095347406802205 ) ;
#37589=VERTEX_POINT ( 'NONE', #59171 ) ;
#37598=ORIENTED_EDGE ( 'NONE', *, *, #19864, .T. ) ;
#37617=VECTOR ( 'NONE', #16121, 1000.000000000000000 ) ;
#37630=DIRECTION ( 'NONE',  ( 0.000000000000000000, 0.000000000000000000, -1.000000000000000000 ) ) ;
#37643=DIRECTION ( 'NONE',  ( 0.000000000000000000, -1.000000000000000000, 0.000000000000000000 ) ) ;
#37651=VECTOR ( 'NONE', #62059, 1000.000000000000000 ) ;
#37667=DIRECTION ( 'NONE',  ( -1.000000000000000000, 0.000000000000000000, 0.000000000000000000 ) ) ;
#37677=EDGE_CURVE ( 'NONE', #16122, #58159, #23305, .T. ) ;
#37714=DIRECTION ( 'NONE',  ( 0.000000000000000000, -0.000000000000000000, -1.000000000000000000 ) ) ;
#37716=DIRECTION ( 'NONE',  ( -0.000000000000000000, -0.000000000000000000, 1.000000000000000000 ) ) ;
#37717=DIRECTION ( 'NONE',  ( -0.000000000000000000, -0.000000000000000000, -1.000000000000000000 ) ) ;
#37718=LINE ( 'NONE', #47920, #23934 ) ;
#37720=AXIS2_PLACEMENT_3D ( 'NONE', #46853, #69340, #21162 ) ;
#37724=EDGE_CURVE ( 'NONE', #37473, #59570, #39136, .T. ) ;
#37725=ORIENTED_EDGE ( 'NONE', *, *, #61365, .F. ) ;
#37742=DIRECTION ( 'NONE',  ( 1.000000000000000000, -0.000000000000000000, -0.000000000000000000 ) ) ;
#37774=ORIENTED_EDGE ( 'NONE', *, *, #4372, .T. ) ;
#37786=EDGE_LOOP ( 'NONE', ( #68093, #30165, #43689, #5755, #69161, #66499, #28331, #63358, #29886, #16583 ) ) ;
#37790=EDGE_CURVE ( 'NONE', #65005, #43260, #13436, .T. ) ;
#37793=EDGE_CURVE ( 'NONE', #45595, #57264, #38368, .T. ) ;
#37810=DIRECTION ( 'NONE',  ( 0.000000000000000000, 1.000000000000000000, 0.000000000000000000 ) ) ;
#37836=CARTESIAN_POINT ( 'NONE',  ( 188.9999999999999432, 0.000000000000000000, 72.99999999999998579 ) ) ;
#37840=CARTESIAN_POINT ( 'NONE',  ( 410.0000000000000000, 0.000000000000000000, 174.3129005282752928 ) ) ;
#37863=CARTESIAN_POINT ( 'NONE',  ( 266.9165763529819628, 192.0000000000000000, 128.9999999999999716 ) ) ;
#37872=CARTESIAN_POINT ( 'NONE',  ( 444.9999999999999432, -35.00000000000000000, -2.000000000000000000 ) ) ;
#37878=AXIS2_PLACEMENT_3D ( 'NONE', #55412, #45211, #44522 ) ;
#37889=CARTESIAN_POINT ( 'NONE',  ( 266.9165763529819628, -2.000000000000001776, 108.9999999999999858 ) ) ;
#37900=CARTESIAN_POINT ( 'NONE',  ( 0.000000000000000000, -2.000000000000000000, 378.0000000000000000 ) ) ;
#37906=CARTESIAN_POINT ( 'NONE',  ( 412.0000000000000000, 192.0000000000000000, 0.000000000000000000 ) ) ;
#37916=VECTOR ( 'NONE', #55721, 1000.000000000000000 ) ;
#37926=ORIENTED_EDGE ( 'NONE', *, *, #46146, .F. ) ;
#37929=DIRECTION ( 'NONE',  ( 0.000000000000000000, 0.000000000000000000, -1.000000000000000000 ) ) ;
#37937=VERTEX_POINT ( 'NONE', #4947 ) ;
#37967=ORIENTED_EDGE ( 'NONE', *, *, #21372, .T. ) ;
#37970=ORIENTED_EDGE ( 'NONE', *, *, #64818, .T. ) ;
#37983=PLANE ( 'NONE',  #24528 ) ;
#37990=DIRECTION ( 'NONE',  ( 0.000000000000000000, 0.000000000000000000, 1.000000000000000000 ) ) ;
#37995=CARTESIAN_POINT ( 'NONE',  ( 432.4999999999999432, -18.06806526123148160, 378.0000000000000000 ) ) ;
#38008=VECTOR ( 'NONE', #12609, 1000.000000000000000 ) ;
#38022=CARTESIAN_POINT ( 'NONE',  ( -22.50000000000003197, 207.5000000000000284, 0.000000000000000000 ) ) ;
#38037=ORIENTED_EDGE ( 'NONE', *, *, #33051, .T. ) ;
#38054=VECTOR ( 'NONE', #12147, 1000.000000000000000 ) ;
#38059=PLANE ( 'NONE',  #61474 ) ;
#38064=DIRECTION ( 'NONE',  ( 0.000000000000000000, 1.000000000000000000, -0.000000000000000000 ) ) ;
#38077=ORIENTED_EDGE ( 'NONE', *, *, #66408, .T. ) ;
#38096=LINE ( 'NONE', #10327, #23982 ) ;
#38102=EDGE_LOOP ( 'NONE', ( #67279, #19344, #35939, #8203, #1696, #30074, #12632, #38928, #34964, #35501 ) ) ;
#38117=VERTEX_POINT ( 'NONE', #29188 ) ;
#38126=LINE ( 'NONE', #59568, #59517 ) ;
#38131=DIRECTION ( 'NONE',  ( 0.000000000000000000, -1.000000000000000000, 0.000000000000000000 ) ) ;
#38136=AXIS2_PLACEMENT_3D ( 'NONE', #28528, #50336, #66188 ) ;
#38186=ORIENTED_EDGE ( 'NONE', *, *, #44865, .T. ) ;
#38225=LINE ( 'NONE', #5521, #51760 ) ;
#38239=AXIS2_PLACEMENT_3D ( 'NONE', #29844, #13666, #56577 ) ;
#38259=EDGE_CURVE ( 'NONE', #59483, #54103, #60920, .T. ) ;
#38269=DIRECTION ( 'NONE',  ( 0.000000000000000000, 1.000000000000000000, 0.000000000000000000 ) ) ;
#38280=ORIENTED_EDGE ( 'NONE', *, *, #37038, .T. ) ;
#38366=DIRECTION ( 'NONE',  ( -0.000000000000000000, -0.000000000000000000, -1.000000000000000000 ) ) ;
#38368=CIRCLE ( 'NONE', #17016, 5.000000000000000888 ) ;
#38374=LINE ( 'NONE', #53500, #31211 ) ;
#38386=DIRECTION ( 'NONE',  ( -0.000000000000000000, -1.000000000000000000, -0.000000000000000000 ) ) ;
#38408=FACE_OUTER_BOUND ( 'NONE', #54498, .T. ) ;
#38475=PLANE ( 'NONE',  #17757 ) ;
#38476=CARTESIAN_POINT ( 'NONE',  ( 144.4165763529819344, 225.8585178651493663, 129.0000000000000000 ) ) ;
#38510=ORIENTED_EDGE ( 'NONE', *, *, #15301, .T. ) ;
#38514=EDGE_LOOP ( 'NONE', ( #29159, #37926 ) ) ;
#38515=VECTOR ( 'NONE', #35394, 1000.000000000000000 ) ;
#38544=FACE_OUTER_BOUND ( 'NONE', #36176, .T. ) ;
#38562=ORIENTED_EDGE ( 'NONE', *, *, #59931, .F. ) ;
#38584=EDGE_CURVE ( 'NONE', #9181, #40644, #27216, .T. ) ;
#38630=VECTOR ( 'NONE', #64814, 1000.000000000000000 ) ;
#38663=DIRECTION ( 'NONE',  ( -1.000000000000000000, -0.000000000000000000, -0.000000000000000000 ) ) ;
#38668=EDGE_CURVE ( 'NONE', #50651, #52456, #58245, .T. ) ;
#38701=ADVANCED_FACE ( 'NONE', ( #4777, #58579, #58926 ), #26247, .F. ) ;
#38713=VERTEX_POINT ( 'NONE', #53646 ) ;
#38720=DIRECTION ( 'NONE',  ( 0.000000000000000000, 0.000000000000000000, -1.000000000000000000 ) ) ;
#38729=AXIS2_PLACEMENT_3D ( 'NONE', #25963, #35830, #9439 ) ;
#38759=EDGE_CURVE ( 'NONE', #27523, #38117, #185, .T. ) ;
#38829=AXIS2_PLACEMENT_3D ( 'NONE', #9486, #68233, #13718 ) ;
#38835=CIRCLE ( 'NONE', #21942, 5.000000000000000888 ) ;
#38843=ORIENTED_EDGE ( 'NONE', *, *, #48079, .F. ) ;
#38896=CARTESIAN_POINT ( 'NONE',  ( 111.9975424824652634, 20.00000000000003197, 401.6295345748407613 ) ) ;
#38928=ORIENTED_EDGE ( 'NONE', *, *, #39192, .T. ) ;
#38956=CARTESIAN_POINT ( 'NONE',  ( 109.9975424824652777, 296.0000000000000000, 418.0000000000000000 ) ) ;
#38973=ADVANCED_FACE ( 'NONE', ( #30661, #14137, #26419 ), #58411, .T. ) ;
#38975=ORIENTED_EDGE ( 'NONE', *, *, #64965, .T. ) ;
#38985=LINE ( 'NONE', #44237, #60871 ) ;
#38987=ORIENTED_EDGE ( 'NONE', *, *, #23377, .T. ) ;
#38988=VECTOR ( 'NONE', #30973, 1000.000000000000000 ) ;
#39001=CARTESIAN_POINT ( 'NONE',  ( 311.9975424824652350, 170.0000000000000284, 354.1673509436691347 ) ) ;
#39008=ORIENTED_EDGE ( 'NONE', *, *, #8036, .F. ) ;
#39034=ORIENTED_EDGE ( 'NONE', *, *, #356, .T. ) ;
#39050=VERTEX_POINT ( 'NONE', #6691 ) ;
#39059=DIRECTION ( 'NONE',  ( -1.240128853613758897E-16, 0.000000000000000000, 1.000000000000000000 ) ) ;
#39067=ORIENTED_EDGE ( 'NONE', *, *, #26906, .T. ) ;
#39071=ADVANCED_FACE ( 'NONE', ( #55219 ), #2809, .F. ) ;
#39073=VECTOR ( 'NONE', #44994, 1000.000000000000000 ) ;
#39086=EDGE_CURVE ( 'NONE', #55507, #68666, #61202, .T. ) ;
#39087=CARTESIAN_POINT ( 'NONE',  ( 444.9999999999999432, 225.0000000000000000, 380.0000000000000000 ) ) ;
#39093=DIRECTION ( 'NONE',  ( -2.509494923690479143E-16, -1.000000000000000000, -1.496132621402170665E-16 ) ) ;
#39105=ADVANCED_FACE ( 'NONE', ( #13027 ), #7396, .F. ) ;
#39108=CARTESIAN_POINT ( 'NONE',  ( 230.9999999999999432, 0.000000000000000000, 72.99999999999998579 ) ) ;
#39110=EDGE_CURVE ( 'NONE', #56653, #31511, #45367, .T. ) ;
#39136=LINE ( 'NONE', #39467, #33921 ) ;
#39138=CARTESIAN_POINT ( 'NONE',  ( 432.4999999999999432, -18.06806526123148160, 0.000000000000000000 ) ) ;
#39140=CARTESIAN_POINT ( 'NONE',  ( -22.50000000000003197, -18.06806526123148160, -2.000000000000000000 ) ) ;
#39146=CARTESIAN_POINT ( 'NONE',  ( 213.7150814747576817, 0.000000000000000000, 277.7615984639418798 ) ) ;
#39191=CARTESIAN_POINT ( 'NONE',  ( 444.9999999999999432, 225.0000000000000000, 0.000000000000000000 ) ) ;
#39192=EDGE_CURVE ( 'NONE', #38713, #26166, #49441, .T. ) ;
#39241=LINE ( 'NONE', #6164, #60369 ) ;
#39245=EDGE_CURVE ( 'NONE', #41662, #13740, #57430, .T. ) ;
#39267=CARTESIAN_POINT ( 'NONE',  ( 311.9975424824652350, 296.0000000000000000, 420.0000000000000000 ) ) ;
#39272=EDGE_CURVE ( 'NONE', #65661, #13467, #39682, .T. ) ;
#39275=ORIENTED_EDGE ( 'NONE', *, *, #37038, .F. ) ;
#39291=DIRECTION ( 'NONE',  ( 0.000000000000000000, 1.000000000000000000, 0.000000000000000000 ) ) ;
#39301=LINE ( 'NONE', #55828, #32145 ) ;
#39362=EDGE_CURVE ( 'NONE', #51848, #37385, #57777, .T. ) ;
#39385=CARTESIAN_POINT ( 'NONE',  ( 313.9975424824652350, 296.0000000000000000, 529.9060149868646477 ) ) ;
#39397=VECTOR ( 'NONE', #64392, 1000.000000000000000 ) ;
#39398=DIRECTION ( 'NONE',  ( 0.000000000000000000, 1.000000000000000000, -0.000000000000000000 ) ) ;
#39407=ORIENTED_EDGE ( 'NONE', *, *, #69004, .T. ) ;
#39441=CIRCLE ( 'NONE', #22613, 5.000000000000004441 ) ;
#39447=DIRECTION ( 'NONE',  ( 0.008343357611899119078, 0.000000000000000000, 0.9999651935861366692 ) ) ;
#39463=EDGE_CURVE ( 'NONE', #60279, #1408, #15558, .T. ) ;
#39465=VERTEX_POINT ( 'NONE', #53512 ) ;
#39467=CARTESIAN_POINT ( 'NONE',  ( 444.9999999999999432, -35.00000000000000000, 378.0000000000000000 ) ) ;
#39498=AXIS2_PLACEMENT_3D ( 'NONE', #18143, #44156, #32919 ) ;
#39501=DIRECTION ( 'NONE',  ( 0.000000000000000000, -1.000000000000000000, 0.000000000000000000 ) ) ;
#39516=CARTESIAN_POINT ( 'NONE',  ( 111.9975424824653487, 18.00000000000002842, 256.6193948016162381 ) ) ;
#39532=ORIENTED_EDGE ( 'NONE', *, *, #68515, .F. ) ;
#39551=ADVANCED_FACE ( 'NONE', ( #63050 ), #41937, .F. ) ;
#39559=CARTESIAN_POINT ( 'NONE',  ( 264.4165763529819628, -27.00000000000000355, 138.9999999999999716 ) ) ;
#39603=ORIENTED_EDGE ( 'NONE', *, *, #15240, .F. ) ;
#39627=CARTESIAN_POINT ( 'NONE',  ( 311.9975424824652350, 20.00000000000003197, 256.6193948016162381 ) ) ;
#39640=LINE ( 'NONE', #38956, #66680 ) ;
#39652=CARTESIAN_POINT ( 'NONE',  ( -35.00000000000002842, -35.00000000000000000, 380.0000000000000000 ) ) ;
#39662=LINE ( 'NONE', #12942, #50800 ) ;
#39670=CARTESIAN_POINT ( 'NONE',  ( 141.9165763529819344, 242.0000000000000000, 108.9999999999999858 ) ) ;
#39682=CIRCLE ( 'NONE', #66671, 5.000000000000000888 ) ;
#39683=CARTESIAN_POINT ( 'NONE',  ( -2.000000000000000000, -2.000000000000000000, 380.0000000000000000 ) ) ;
#39702=FACE_OUTER_BOUND ( 'NONE', #7592, .T. ) ;
#39705=LINE ( 'NONE', #23534, #25542 ) ;
#39709=LINE ( 'NONE', #23540, #53530 ) ;
#39713=EDGE_LOOP ( 'NONE', ( #52115, #19097, #36125, #39815 ) ) ;
#39722=EDGE_CURVE ( 'NONE', #5460, #31511, #55391, .T. ) ;
#39796=ORIENTED_EDGE ( 'NONE', *, *, #52932, .T. ) ;
#39815=ORIENTED_EDGE ( 'NONE', *, *, #22530, .F. ) ;
#39823=CYLINDRICAL_SURFACE ( 'NONE', #2229, 5.000000000000004441 ) ;
#39839=CIRCLE ( 'NONE', #3895, 21.00000000000000355 ) ;
#39843=VECTOR ( 'NONE', #46226, 1000.000000000000000 ) ;
#39894=CARTESIAN_POINT ( 'NONE',  ( 111.9975424824652634, 296.0000000000000000, 529.9060149868646477 ) ) ;
#39901=ORIENTED_EDGE ( 'NONE', *, *, #54213, .T. ) ;
#39904=CARTESIAN_POINT ( 'NONE',  ( 209.3223706822284100, 0.000000000000000000, 276.7520087653757628 ) ) ;
#39905=CARTESIAN_POINT ( 'NONE',  ( 410.0000000000000000, 190.0000000000000000, 174.3129005282752928 ) ) ;
#39921=CARTESIAN_POINT ( 'NONE',  ( 311.9975424824652350, 20.00000000000003197, 256.6193948016162381 ) ) ;
#39925=EDGE_CURVE ( 'NONE', #44925, #20626, #8261, .T. ) ;
#39926=AXIS2_PLACEMENT_3D ( 'NONE', #17336, #39501, #1165 ) ;
#39948=ORIENTED_EDGE ( 'NONE', *, *, #17132, .F. ) ;
#39959=ORIENTED_EDGE ( 'NONE', *, *, #42105, .T. ) ;
#39973=ORIENTED_EDGE ( 'NONE', *, *, #69243, .T. ) ;
#39982=AXIS2_PLACEMENT_3D ( 'NONE', #62945, #67891, #61567 ) ;
#39992=VECTOR ( 'NONE', #65518, 1000.000000000000000 ) ;
#40005=ORIENTED_EDGE ( 'NONE', *, *, #22530, .T. ) ;
#40029=ORIENTED_EDGE ( 'NONE', *, *, #19360, .T. ) ;
#40030=EDGE_CURVE ( 'NONE', #56454, #18878, #37453, .T. ) ;
#40038=CARTESIAN_POINT ( 'NONE',  ( -17.50000000000002842, 207.5000000000000284, 0.000000000000000000 ) ) ;
#40081=VECTOR ( 'NONE', #41597, 1000.000000000000000 ) ;
#40102=ORIENTED_EDGE ( 'NONE', *, *, #45999, .F. ) ;
#40114=EDGE_CURVE ( 'NONE', #59570, #47824, #19983, .T. ) ;
#40125=AXIS2_PLACEMENT_3D ( 'NONE', #16459, #53729, #6244 ) ;
#40144=VECTOR ( 'NONE', #14446, 1000.000000000000000 ) ;
#40153=CIRCLE ( 'NONE', #37878, 246.3582898394606957 ) ;
#40156=VERTEX_POINT ( 'NONE', #11136 ) ;
#40174=EDGE_CURVE ( 'NONE', #36497, #43728, #22042, .T. ) ;
#40191=DIRECTION ( 'NONE',  ( -1.000000000000000000, 0.000000000000000000, 0.000000000000000000 ) ) ;
#40194=AXIS2_PLACEMENT_3D ( 'NONE', #43472, #33298, #21678 ) ;
#40223=CIRCLE ( 'NONE', #61562, 5.000000000000004441 ) ;
#40314=LINE ( 'NONE', #23461, #21412 ) ;
#40320=CARTESIAN_POINT ( 'NONE',  ( -35.00000000000002842, 225.0000000000000000, 0.000000000000000000 ) ) ;
#40338=DIRECTION ( 'NONE',  ( -1.000000000000000000, 0.000000000000000000, 0.000000000000000000 ) ) ;
#40346=DIRECTION ( 'NONE',  ( 2.220446049250313081E-16, 0.000000000000000000, 1.000000000000000000 ) ) ;
#40354=VERTEX_POINT ( 'NONE', #25184 ) ;
#40365=EDGE_CURVE ( 'NONE', #1408, #52352, #68095, .T. ) ;
#40403=CARTESIAN_POINT ( 'NONE',  ( 266.9165763529819628, 242.0000000000000000, 128.9999999999999716 ) ) ;
#40443=FACE_OUTER_BOUND ( 'NONE', #28989, .T. ) ;
#40496=CARTESIAN_POINT ( 'NONE',  ( 141.9165763529819344, 242.0000000000000000, 129.0000000000000000 ) ) ;
#40500=ORIENTED_EDGE ( 'NONE', *, *, #49772, .T. ) ;
#40513=CARTESIAN_POINT ( 'NONE',  ( 141.9165763529819344, 242.0000000000000000, 108.9999999999999858 ) ) ;
#40535=AXIS2_PLACEMENT_3D ( 'NONE', #6043, #43327, #37714 ) ;
#40546=DIRECTION ( 'NONE',  ( -0.000000000000000000, -0.000000000000000000, -1.000000000000000000 ) ) ;
#40582=ADVANCED_FACE ( 'NONE', ( #47222 ), #69017, .F. ) ;
#40608=CARTESIAN_POINT ( 'NONE',  ( 111.9975424824652634, 170.0000000000000284, 536.6193948016162949 ) ) ;
#40621=DIRECTION ( 'NONE',  ( 0.000000000000000000, -0.000000000000000000, -1.000000000000000000 ) ) ;
#40634=DIRECTION ( 'NONE',  ( 0.000000000000000000, -1.000000000000000000, -0.000000000000000000 ) ) ;
#40644=VERTEX_POINT ( 'NONE', #47558 ) ;
#40668=ORIENTED_EDGE ( 'NONE', *, *, #32393, .T. ) ;
#40672=CARTESIAN_POINT ( 'NONE',  ( 444.9999999999999432, -35.00000000000000000, -2.000000000000000000 ) ) ;
#40686=CIRCLE ( 'NONE', #45159, 5.000000000000004441 ) ;
#40700=AXIS2_PLACEMENT_3D ( 'NONE', #59364, #43530, #54784 ) ;
#40724=ORIENTED_EDGE ( 'NONE', *, *, #59581, .T. ) ;
#40730=VERTEX_POINT ( 'NONE', #55534 ) ;
#40737=VECTOR ( 'NONE', #16372, 1000.000000000000000 ) ;
#40746=LINE ( 'NONE', #61847, #51042 ) ;
#40787=AXIS2_PLACEMENT_3D ( 'NONE', #18498, #33299, #13231 ) ;
#40852=ORIENTED_EDGE ( 'NONE', *, *, #39245, .F. ) ;
#40880=FACE_OUTER_BOUND ( 'NONE', #23853, .T. ) ;
#40882=LINE ( 'NONE', #13466, #24287 ) ;
#40915=CARTESIAN_POINT ( 'NONE',  ( 444.9999999999999432, -35.00000000000000000, 380.0000000000000000 ) ) ;
#40978=CARTESIAN_POINT ( 'NONE',  ( 422.4999999999999432, -18.06806526123148160, 0.000000000000000000 ) ) ;
#40983=VECTOR ( 'NONE', #30092, 1000.000000000000000 ) ;
#40994=DIRECTION ( 'NONE',  ( -1.000000000000000000, 0.000000000000000000, 0.000000000000000000 ) ) ;
#41018=CARTESIAN_POINT ( 'NONE',  ( 311.9975424824652350, 296.0000000000000000, 420.0000000000000000 ) ) ;
#41029=ORIENTED_EDGE ( 'NONE', *, *, #33633, .T. ) ;
#41067=CARTESIAN_POINT ( 'NONE',  ( 109.9975424824652634, 171.8183490441642789, 533.9018882243741473 ) ) ;
#41069=EDGE_CURVE ( 'NONE', #12143, #56454, #22055, .T. ) ;
#41070=ORIENTED_EDGE ( 'NONE', *, *, #13596, .F. ) ;
#41172=CYLINDRICAL_SURFACE ( 'NONE', #9418, 164.5210298272983778 ) ;
#41180=VERTEX_POINT ( 'NONE', #40320 ) ;
#41212=DIRECTION ( 'NONE',  ( 0.000000000000000000, 0.000000000000000000, 1.000000000000000000 ) ) ;
#41296=AXIS2_PLACEMENT_3D ( 'NONE', #43974, #38720, #60166 ) ;
#41323=CARTESIAN_POINT ( 'NONE',  ( 209.3223706822284100, 172.0000000000000284, 31.44247402469554942 ) ) ;
#41328=ORIENTED_EDGE ( 'NONE', *, *, #44105, .F. ) ;
#41382=EDGE_LOOP ( 'NONE', ( #58703, #48312, #64394, #401 ) ) ;
#41389=ADVANCED_FACE ( 'NONE', ( #56074 ), #33930, .F. ) ;
#41433=CARTESIAN_POINT ( 'NONE',  ( 209.3223706822284100, 190.0000000000000000, 31.44247402469554942 ) ) ;
#41448=VERTEX_POINT ( 'NONE', #67336 ) ;
#41466=EDGE_LOOP ( 'NONE', ( #22509, #65412, #47155, #60647 ) ) ;
#41543=ADVANCED_FACE ( 'NONE', ( #33504 ), #44025, .T. ) ;
#41565=CARTESIAN_POINT ( 'NONE',  ( 188.9999999999999432, -57.00000000000007816, 72.99999999999998579 ) ) ;
#41573=CARTESIAN_POINT ( 'NONE',  ( 111.9975424824652634, 296.0000000000000000, 420.0000000000000568 ) ) ;
#41587=DIRECTION ( 'NONE',  ( 0.000000000000000000, 1.000000000000000000, 0.000000000000000000 ) ) ;
#41588=ADVANCED_FACE ( 'NONE', ( #47918 ), #17302, .F. ) ;
#41597=DIRECTION ( 'NONE',  ( 1.000000000000000000, -0.000000000000000000, -0.000000000000000000 ) ) ;
#41614=AXIS2_PLACEMENT_3D ( 'NONE', #35823, #57277, #44183 ) ;
#41628=CARTESIAN_POINT ( 'NONE',  ( 111.9975424824652634, 172.0000000000000284, 420.0000000000000568 ) ) ;
#41637=ORIENTED_EDGE ( 'NONE', *, *, #58353, .T. ) ;
#41662=VERTEX_POINT ( 'NONE', #45783 ) ;
#41687=ADVANCED_FACE ( 'NONE', ( #60566 ), #13766, .F. ) ;
#41690=EDGE_LOOP ( 'NONE', ( #3315, #1023, #40500, #65521, #62901, #5058, #31975, #55182, #30559, #4992, #37250, #57444 ) ) ;
#41691=EDGE_CURVE ( 'NONE', #32243, #37937, #1477, .T. ) ;
#41696=VECTOR ( 'NONE', #55548, 1000.000000000000000 ) ;
#41736=ORIENTED_EDGE ( 'NONE', *, *, #8036, .T. ) ;
#41766=CARTESIAN_POINT ( 'NONE',  ( 311.9975424824652350, 296.0000000000000000, 420.0000000000000000 ) ) ;
#41812=CARTESIAN_POINT ( 'NONE',  ( -35.00000000000002842, 225.0000000000000000, 378.0000000000000000 ) ) ;
#41816=ORIENTED_EDGE ( 'NONE', *, *, #43792, .F. ) ;
#41831=PLANE ( 'NONE',  #42034 ) ;
#41838=CARTESIAN_POINT ( 'NONE',  ( 188.9999999999999432, -35.00000000000000000, -2.000000000000000000 ) ) ;
#41862=EDGE_CURVE ( 'NONE', #5291, #61739, #47586, .T. ) ;
#41896=AXIS2_PLACEMENT_3D ( 'NONE', #35099, #13994, #63222 ) ;
#41906=ORIENTED_EDGE ( 'NONE', *, *, #27290, .T. ) ;
#41930=CARTESIAN_POINT ( 'NONE',  ( 410.0000000000000000, 190.0000000000000000, 380.0000000000000000 ) ) ;
#41937=CYLINDRICAL_SURFACE ( 'NONE', #20540, 5.000000000000000888 ) ;
#41988=DIRECTION ( 'NONE',  ( 0.000000000000000000, 0.000000000000000000, -1.000000000000000000 ) ) ;
#41994=VECTOR ( 'NONE', #29584, 1000.000000000000000 ) ;
#41996=VECTOR ( 'NONE', #11209, 1000.000000000000000 ) ;
#42006=DIRECTION ( 'NONE',  ( 1.000000000000000000, 0.000000000000000000, 0.000000000000000000 ) ) ;
#42009=AXIS2_PLACEMENT_3D ( 'NONE', #22134, #28102, #43921 ) ;
#42034=AXIS2_PLACEMENT_3D ( 'NONE', #20035, #15100, #25666 ) ;
#42052=ORIENTED_EDGE ( 'NONE', *, *, #51706, .T. ) ;
#42105=EDGE_CURVE ( 'NONE', #7559, #295, #46486, .T. ) ;
#42124=DIRECTION ( 'NONE',  ( -0.000000000000000000, -0.000000000000000000, 1.000000000000000000 ) ) ;
#42190=VECTOR ( 'NONE', #48240, 1000.000000000000000 ) ;
#42194=LINE ( 'NONE', #4559, #9 ) ;
#42199=VECTOR ( 'NONE', #44146, 1000.000000000000000 ) ;
#42213=DIRECTION ( 'NONE',  ( 0.000000000000000000, 1.000000000000000000, 0.000000000000000000 ) ) ;
#42236=VERTEX_POINT ( 'NONE', #33084 ) ;
#42244=AXIS2_PLACEMENT_3D ( 'NONE', #28294, #49387, #2277 ) ;
#42268=DIRECTION ( 'NONE',  ( 0.000000000000000000, 0.000000000000000000, -1.000000000000000000 ) ) ;
#42280=CARTESIAN_POINT ( 'NONE',  ( 209.3223706822284100, 0.000000000000000000, 31.44247402469554942 ) ) ;
#42281=VERTEX_POINT ( 'NONE', #24970 ) ;
#42317=ADVANCED_FACE ( 'NONE', ( #26689, #48118, #14743 ), #41831, .T. ) ;
#42399=ORIENTED_EDGE ( 'NONE', *, *, #46938, .T. ) ;
#42437=CARTESIAN_POINT ( 'NONE',  ( 154.4165763529819628, -26.99999999999998224, 108.9999999999999858 ) ) ;
#42478=VECTOR ( 'NONE', #44290, 1000.000000000000000 ) ;
#42480=ADVANCED_FACE ( 'NONE', ( #28776 ), #23849, .T. ) ;
#42485=CARTESIAN_POINT ( 'NONE',  ( 307.2575771313985342, 18.00000000000002842, 256.6193948016162381 ) ) ;
#42489=VECTOR ( 'NONE', #2135, 1000.000000000000000 ) ;
#42498=EDGE_CURVE ( 'NONE', #20901, #60423, #58888, .T. ) ;
#42513=DIRECTION ( 'NONE',  ( 2.220446049250313081E-16, 0.000000000000000000, 1.000000000000000000 ) ) ;
#42566=ORIENTED_EDGE ( 'NONE', *, *, #12140, .F. ) ;
#42570=CARTESIAN_POINT ( 'NONE',  ( 111.9975424824652634, 296.0000000000000000, 529.9060149868646477 ) ) ;
#42606=FACE_OUTER_BOUND ( 'NONE', #18389, .T. ) ;
#42628=CARTESIAN_POINT ( 'NONE',  ( 412.0000000000000000, -2.000000000000000000, 378.0000000000000000 ) ) ;
#42661=CARTESIAN_POINT ( 'NONE',  ( 230.9999999999999432, 0.000000000000000000, 0.000000000000000000 ) ) ;
#42700=DIRECTION ( 'NONE',  ( 0.000000000000000000, 0.000000000000000000, 1.000000000000000000 ) ) ;
#42703=ORIENTED_EDGE ( 'NONE', *, *, #19360, .F. ) ;
#42741=ORIENTED_EDGE ( 'NONE', *, *, #463, .T. ) ;
#42758=ORIENTED_EDGE ( 'NONE', *, *, #51653, .F. ) ;
#42782=CARTESIAN_POINT ( 'NONE',  ( 427.4999999999999432, 207.5000000000000284, 0.000000000000000000 ) ) ;
#42785=CARTESIAN_POINT ( 'NONE',  ( 230.9999999999999432, 192.0000000000000000, 72.99999999999998579 ) ) ;
#42791=VECTOR ( 'NONE', #60258, 1000.000000000000000 ) ;
#42815=CARTESIAN_POINT ( 'NONE',  ( 311.9975424824652350, 20.00000000000003197, 255.6641978984094408 ) ) ;
#42824=LINE ( 'NONE', #69560, #44751 ) ;
#42850=DIRECTION ( 'NONE',  ( 0.000000000000000000, 0.000000000000000000, -1.000000000000000000 ) ) ;
#42858=LINE ( 'NONE', #39001, #54463 ) ;
#42859=LINE ( 'NONE', #48464, #48135 ) ;
#42862=DIRECTION ( 'NONE',  ( 0.000000000000000000, 0.000000000000000000, -1.000000000000000000 ) ) ;
#42897=DIRECTION ( 'NONE',  ( -0.000000000000000000, -0.000000000000000000, 1.000000000000000000 ) ) ;
#42908=CARTESIAN_POINT ( 'NONE',  ( 412.0000000000000000, -2.000000000000000000, 0.000000000000000000 ) ) ;
#42937=CARTESIAN_POINT ( 'NONE',  ( 141.9165763529819344, -52.00000000000000711, 129.0000000000000000 ) ) ;
#42978=CIRCLE ( 'NONE', #41896, 246.3582898394606957 ) ;
#42984=VECTOR ( 'NONE', #49112, 1000.000000000000000 ) ;
#42999=ADVANCED_FACE ( 'NONE', ( #10503 ), #26694, .F. ) ;
#43001=CARTESIAN_POINT ( 'NONE',  ( 209.3223706822284100, 190.0000000000000000, 276.7520087653757628 ) ) ;
#43019=CARTESIAN_POINT ( 'NONE',  ( 311.9975424824652350, 20.00000000000003197, 380.0000000000001137 ) ) ;
#43030=AXIS2_PLACEMENT_3D ( 'NONE', #7675, #55492, #62775 ) ;
#43074=PRODUCT_CONTEXT ( 'NONE', #14326, 'mechanical' ) ;
#43083=CARTESIAN_POINT ( 'NONE',  ( -35.00000000000002842, -35.00000000000000000, 0.000000000000000000 ) ) ;
#43088=ORIENTED_EDGE ( 'NONE', *, *, #24415, .F. ) ;
#43132=CIRCLE ( 'NONE', #33065, 5.000000000000004441 ) ;
#43171=EDGE_CURVE ( 'NONE', #37385, #63094, #50576, .T. ) ;
#43182=DIRECTION ( 'NONE',  ( -0.000000000000000000, -0.000000000000000000, -1.000000000000000000 ) ) ;
#43192=CARTESIAN_POINT ( 'NONE',  ( 0.000000000000000000, 192.0000000000000000, 0.000000000000000000 ) ) ;
#43204=CARTESIAN_POINT ( 'NONE',  ( 141.9165763529819344, 242.0000000000000000, 129.0000000000000000 ) ) ;
#43227=CARTESIAN_POINT ( 'NONE',  ( 154.4165763529819628, -26.99999999999998224, 129.0000000000000000 ) ) ;
#43260=VERTEX_POINT ( 'NONE', #44527 ) ;
#43261=AXIS2_PLACEMENT_3D ( 'NONE', #67211, #2821, #52047 ) ;
#43275=AXIS2_PLACEMENT_3D ( 'NONE', #27546, #48986, #60953 ) ;
#43292=CARTESIAN_POINT ( 'NONE',  ( 412.0000000000000000, 0.000000000000000000, -0.000000000000000000 ) ) ;
#43316=EDGE_CURVE ( 'NONE', #11641, #49852, #5832, .T. ) ;
#43321=CARTESIAN_POINT ( 'NONE',  ( 427.4999999999999432, -18.06806526123148160, 380.0000000000000000 ) ) ;
#43327=DIRECTION ( 'NONE',  ( 0.000000000000000000, -1.000000000000000000, 0.000000000000000000 ) ) ;
#43366=ORIENTED_EDGE ( 'NONE', *, *, #58511, .F. ) ;
#43375=ORIENTED_EDGE ( 'NONE', *, *, #35171, .T. ) ;
#43378=VERTEX_POINT ( 'NONE', #10014 ) ;
#43441=DIRECTION ( 'NONE',  ( 0.000000000000000000, 1.000000000000000000, 0.000000000000000000 ) ) ;
#43467=ORIENTED_EDGE ( 'NONE', *, *, #40030, .T. ) ;
#43472=CARTESIAN_POINT ( 'NONE',  ( 209.9518228411288874, 170.0000000000000284, 31.43423095485942298 ) ) ;
#43488=EDGE_CURVE ( 'NONE', #13467, #65661, #46597, .T. ) ;
#43526=CARTESIAN_POINT ( 'NONE',  ( -12.50000000000002842, 207.5000000000000284, 380.0000000000000000 ) ) ;
#43530=DIRECTION ( 'NONE',  ( 0.000000000000000000, 0.000000000000000000, 1.000000000000000000 ) ) ;
#43553=ADVANCED_FACE ( 'NONE', ( #11728 ), #43727, .T. ) ;
#43558=LINE ( 'NONE', #53416, #26943 ) ;
#43592=ADVANCED_FACE ( 'NONE', ( #13480 ), #56737, .F. ) ;
#43596=ORIENTED_EDGE ( 'NONE', *, *, #43981, .F. ) ;
#43669=PRODUCT_DEFINITION_CONTEXT ( 'detailed design', #44923, 'design' ) ;
#43689=ORIENTED_EDGE ( 'NONE', *, *, #18122, .F. ) ;
#43702=FACE_OUTER_BOUND ( 'NONE', #17883, .T. ) ;
#43708=CARTESIAN_POINT ( 'NONE',  ( 311.9975424824652350, 172.0000000000000284, 420.0000000000000000 ) ) ;
#43727=PLANE ( 'NONE',  #57853 ) ;
#43728=VERTEX_POINT ( 'NONE', #51802 ) ;
#43730=ORIENTED_EDGE ( 'NONE', *, *, #1668, .F. ) ;
#43735=ADVANCED_FACE ( 'NONE', ( #20134 ), #3610, .T. ) ;
#43745=LINE ( 'NONE', #44816, #55206 ) ;
#43768=PLANE ( 'NONE',  #55457 ) ;
#43781=CARTESIAN_POINT ( 'NONE',  ( 313.9975424824652350, 295.8720703627916464, 535.5371946177799600 ) ) ;
#43792=EDGE_CURVE ( 'NONE', #12534, #30930, #68167, .T. ) ;
#43843=CARTESIAN_POINT ( 'NONE',  ( 313.9975424824652350, 18.08738615523480675, 402.4289050101931480 ) ) ;
#43853=CIRCLE ( 'NONE', #41614, 21.00000000000000355 ) ;
#43866=FACE_OUTER_BOUND ( 'NONE', #29863, .T. ) ;
#43909=FACE_OUTER_BOUND ( 'NONE', #33708, .T. ) ;
#43921=DIRECTION ( 'NONE',  ( -7.128142269859545174E-15, 0.000000000000000000, 1.000000000000000000 ) ) ;
#43959=EDGE_CURVE ( 'NONE', #14754, #38713, #19154, .T. ) ;
#43974=CARTESIAN_POINT ( 'NONE',  ( 427.4999999999999432, -18.06806526123148160, 0.000000000000000000 ) ) ;
#43981=EDGE_CURVE ( 'NONE', #68666, #22151, #35341, .T. ) ;
#43983=VECTOR ( 'NONE', #65878, 1000.000000000000000 ) ;
#44003=CARTESIAN_POINT ( 'NONE',  ( 432.4999999999999432, 207.5000000000000284, 380.0000000000000000 ) ) ;
#44019=DIRECTION ( 'NONE',  ( -1.000000000000000000, 0.000000000000000000, 0.000000000000000000 ) ) ;
#44025=PLANE ( 'NONE',  #61071 ) ;
#44034=CYLINDRICAL_SURFACE ( 'NONE', #1783, 5.000000000000004441 ) ;
#44044=CIRCLE ( 'NONE', #49667, 5.000000000000004441 ) ;
#44063=LINE ( 'NONE', #17339, #47268 ) ;
#44082=VECTOR ( 'NONE', #68791, 1000.000000000000000 ) ;
#44084=FACE_OUTER_BOUND ( 'NONE', #50421, .T. ) ;
#44105=EDGE_CURVE ( 'NONE', #14130, #48350, #51132, .T. ) ;
#44127=CARTESIAN_POINT ( 'NONE',  ( 0.000000000000000000, 319.5570082923146060, 14.52694631438418860 ) ) ;
#44146=DIRECTION ( 'NONE',  ( -0.000000000000000000, 1.000000000000000000, -0.000000000000000000 ) ) ;
#44152=ORIENTED_EDGE ( 'NONE', *, *, #36949, .T. ) ;
#44156=DIRECTION ( 'NONE',  ( 0.000000000000000000, -0.9997420440737085912, -0.02271222823333338831 ) ) ;
#44162=EDGE_LOOP ( 'NONE', ( #4247, #60694, #35763, #24178 ) ) ;
#44176=FACE_OUTER_BOUND ( 'NONE', #18552, .T. ) ;
#44183=DIRECTION ( 'NONE',  ( 0.000000000000000000, 0.000000000000000000, 1.000000000000000000 ) ) ;
#44195=CARTESIAN_POINT ( 'NONE',  ( 309.8720357909272707, 20.00000000000003197, 256.6193948016162381 ) ) ;
#44225=CARTESIAN_POINT ( 'NONE',  ( 254.4165763529819344, -27.00000000000000355, 138.9999999999999716 ) ) ;
#44227=ORIENTED_EDGE ( 'NONE', *, *, #49772, .F. ) ;
#44236=EDGE_CURVE ( 'NONE', #29725, #43378, #59804, .T. ) ;
#44237=CARTESIAN_POINT ( 'NONE',  ( 266.9165763529819628, 242.0000000000000000, 128.9999999999999716 ) ) ;
#44252=CIRCLE ( 'NONE', #30664, 5.000000000000004441 ) ;
#44290=DIRECTION ( 'NONE',  ( 1.000000000000000000, -0.000000000000000000, -0.000000000000000000 ) ) ;
#44292=AXIS2_PLACEMENT_3D ( 'NONE', #18955, #13672, #12638 ) ;
#44301=VECTOR ( 'NONE', #43441, 1000.000000000000000 ) ;
#44302=EDGE_CURVE ( 'NONE', #20626, #13843, #34316, .T. ) ;
#44307=PLANE ( 'NONE',  #10924 ) ;
#44372=ADVANCED_FACE ( 'NONE', ( #14063 ), #3862, .F. ) ;
#44384=ADVANCED_FACE ( 'NONE', ( #57675 ), #46765, .F. ) ;
#44396=VECTOR ( 'NONE', #50864, 1000.000000000000000 ) ;
#44400=AXIS2_PLACEMENT_3D ( 'NONE', #27536, #48978, #821 ) ;
#44465=UNCERTAINTY_MEASURE_WITH_UNIT (LENGTH_MEASURE( 1.000000000000000082E-05 ), #3673, 'distance_accuracy_value', 'NONE');
#44466=EDGE_CURVE ( 'NONE', #65444, #20075, #59986, .T. ) ;
#44478=CARTESIAN_POINT ( 'NONE',  ( 211.9975424824651782, -5.943947286559811093E-16, 276.7368757365948113 ) ) ;
#44479=EDGE_CURVE ( 'NONE', #55507, #13050, #64939, .T. ) ;
#44485=LINE ( 'NONE', #55739, #29895 ) ;
#44486=ORIENTED_EDGE ( 'NONE', *, *, #48258, .T. ) ;
#44522=DIRECTION ( 'NONE',  ( 0.000000000000000000, 0.000000000000000000, 1.000000000000000000 ) ) ;
#44527=CARTESIAN_POINT ( 'NONE',  ( 432.4999999999999432, 207.5000000000000284, -2.000000000000000000 ) ) ;
#44534=DIRECTION ( 'NONE',  ( -0.000000000000000000, 1.000000000000000000, -0.000000000000000000 ) ) ;
#44543=DIRECTION ( 'NONE',  ( -0.000000000000000000, -0.000000000000000000, 1.000000000000000000 ) ) ;
#44546=CARTESIAN_POINT ( 'NONE',  ( 109.9975424824652634, 295.6904194069557548, 539.5330678552892323 ) ) ;
#44558=DIRECTION ( 'NONE',  ( 0.000000000000000000, 0.000000000000000000, 1.000000000000000000 ) ) ;
#44560=CARTESIAN_POINT ( 'NONE',  ( 209.3223706822284100, -1.426547569622074412E-15, 276.7520087653757628 ) ) ;
#44564=CARTESIAN_POINT ( 'NONE',  ( 311.9975424824652350, 170.0000000000000284, 401.6295345748407613 ) ) ;
#44642=LINE ( 'NONE', #22486, #13983 ) ;
#44645=ORIENTED_EDGE ( 'NONE', *, *, #3263, .T. ) ;
#44660=STYLED_ITEM ( 'NONE', ( #52883 ), #62812 ) ;
#44666=CIRCLE ( 'NONE', #41296, 5.000000000000004441 ) ;
#44689=LINE ( 'NONE', #66167, #19961 ) ;
#44720=EDGE_CURVE ( 'NONE', #20626, #26255, #33974, .T. ) ;
#44737=CARTESIAN_POINT ( 'NONE',  ( 109.9975424824652634, 172.0000000000000284, 536.6193948016162949 ) ) ;
#44751=VECTOR ( 'NONE', #20693, 1000.000000000000000 ) ;
#44753=DIRECTION ( 'NONE',  ( -0.000000000000000000, -0.000000000000000000, -1.000000000000000000 ) ) ;
#44768=VERTEX_POINT ( 'NONE', #66354 ) ;
#44802=VECTOR ( 'NONE', #29709, 1000.000000000000000 ) ;
#44816=CARTESIAN_POINT ( 'NONE',  ( 313.9975424824652350, 170.0000000000000284, 256.6193948016162381 ) ) ;
#44849=LINE ( 'NONE', #66333, #39843 ) ;
#44856=VERTEX_POINT ( 'NONE', #20904 ) ;
#44865=EDGE_CURVE ( 'NONE', #31241, #16169, #51875, .T. ) ;
#44879=ORIENTED_EDGE ( 'NONE', *, *, #33196, .T. ) ;
#44892=LINE ( 'NONE', #44546, #47600 ) ;
#44905=CARTESIAN_POINT ( 'NONE',  ( 410.0000000000000000, 190.0000000000000000, -2.000000000000000000 ) ) ;
#44921=DIRECTION ( 'NONE',  ( -2.509494923690479143E-16, -1.000000000000000000, -1.496132621402170665E-16 ) ) ;
#44923=APPLICATION_CONTEXT ( 'automotive_design' ) ;
#44925=VERTEX_POINT ( 'NONE', #48638 ) ;
#44942=CARTESIAN_POINT ( 'NONE',  ( 209.3223706822284100, -1.426547569622074412E-15, 31.44247402469554942 ) ) ;
#44945=VECTOR ( 'NONE', #29444, 1000.000000000000000 ) ;
#44955=EDGE_LOOP ( 'NONE', ( #18758, #31447, #28124, #37967 ) ) ;
#44971=CARTESIAN_POINT ( 'NONE',  ( 209.3223706822284100, 0.000000000000000000, 31.44247402469554942 ) ) ;
#44973=DIRECTION ( 'NONE',  ( -1.000000000000000000, 0.000000000000000000, 0.000000000000000000 ) ) ;
#44985=LINE ( 'NONE', #24593, #7257 ) ;
#44994=DIRECTION ( 'NONE',  ( -0.000000000000000000, -0.000000000000000000, 1.000000000000000000 ) ) ;
#45002=DIRECTION ( 'NONE',  ( -0.000000000000000000, 0.02271222823333339177, -0.9997420440737084801 ) ) ;
#45009=ORIENTED_EDGE ( 'NONE', *, *, #56695, .F. ) ;
#45022=DIRECTION ( 'NONE',  ( -1.000000000000000000, 0.000000000000000000, 0.000000000000000000 ) ) ;
#45038=EDGE_CURVE ( 'NONE', #51213, #8603, #33254, .T. ) ;
#45053=CARTESIAN_POINT ( 'NONE',  ( 209.9518228411288874, 18.00000000000002842, 31.43423095485942298 ) ) ;
#45068=VECTOR ( 'NONE', #35468, 1000.000000000000000 ) ;
#45078=CARTESIAN_POINT ( 'NONE',  ( 313.9975424824652350, 295.6904194069557548, 539.5330678552892323 ) ) ;
#45119=ORIENTED_EDGE ( 'NONE', *, *, #64817, .T. ) ;
#45132=DIRECTION ( 'NONE',  ( -1.000000000000000000, 0.000000000000000000, -0.000000000000000000 ) ) ;
#45153=CYLINDRICAL_SURFACE ( 'NONE', #10218, 5.000000000000004441 ) ;
#45159=AXIS2_PLACEMENT_3D ( 'NONE', #51442, #30672, #40191 ) ;
#45179=EDGE_LOOP ( 'NONE', ( #19109, #3659 ) ) ;
#45190=VERTEX_POINT ( 'NONE', #45826 ) ;
#45211=DIRECTION ( 'NONE',  ( -0.000000000000000000, 1.000000000000000000, 0.000000000000000000 ) ) ;
#45240=LINE ( 'NONE', #66034, #23648 ) ;
#45244=ORIENTED_EDGE ( 'NONE', *, *, #21045, .T. ) ;
#45253=EDGE_CURVE ( 'NONE', #536, #27491, #18696, .T. ) ;
#45266=DIRECTION ( 'NONE',  ( -0.000000000000000000, -0.000000000000000000, 1.000000000000000000 ) ) ;
#45367=LINE ( 'NONE', #18636, #5913 ) ;
#45436=DIRECTION ( 'NONE',  ( -0.000000000000000000, -1.000000000000000000, 0.000000000000000000 ) ) ;
#45443=FACE_BOUND ( 'NONE', #36363, .T. ) ;
#45448=AXIS2_PLACEMENT_3D ( 'NONE', #31972, #42850, #48126 ) ;
#45453=ORIENTED_EDGE ( 'NONE', *, *, #48905, .F. ) ;
#45473=EDGE_CURVE ( 'NONE', #28668, #44925, #17622, .T. ) ;
#45564=DIRECTION ( 'NONE',  ( 0.000000000000000000, -1.000000000000000000, -2.921639538487254261E-16 ) ) ;
#45584=LINE ( 'NONE', #17096, #7154 ) ;
#45593=LINE ( 'NONE', #2687, #37164 ) ;
#45594=LINE ( 'NONE', #39627, #15139 ) ;
#45595=VERTEX_POINT ( 'NONE', #3521 ) ;
#45611=DIRECTION ( 'NONE',  ( -0.000000000000000000, -1.000000000000000000, -0.000000000000000000 ) ) ;
#45635=VERTEX_POINT ( 'NONE', #63311 ) ;
#45647=ORIENTED_EDGE ( 'NONE', *, *, #10938, .T. ) ;
#45657=ORIENTED_EDGE ( 'NONE', *, *, #68920, .F. ) ;
#45675=EDGE_CURVE ( 'NONE', #11610, #69411, #15465, .T. ) ;
#45690=EDGE_LOOP ( 'NONE', ( #42758, #46484, #68234, #15113 ) ) ;
#45745=CARTESIAN_POINT ( 'NONE',  ( 209.9518228411288874, 190.0000000000000000, 31.43423095485942298 ) ) ;
#45783=CARTESIAN_POINT ( 'NONE',  ( 0.000000000000000000, 0.000000000000000000, 380.0000000000000000 ) ) ;
#45826=CARTESIAN_POINT ( 'NONE',  ( 410.0000000000000000, 0.000000000000000000, 380.0000000000000000 ) ) ;
#45838=EDGE_CURVE ( 'NONE', #22362, #56285, #32195, .T. ) ;
#45888=ORIENTED_EDGE ( 'NONE', *, *, #46938, .F. ) ;
#45905=CARTESIAN_POINT ( 'NONE',  ( -22.50000000000003197, 207.5000000000000284, 378.0000000000000000 ) ) ;
#45953=DIRECTION ( 'NONE',  ( -1.000000000000000000, 0.000000000000000000, 0.000000000000000000 ) ) ;
#45955=CARTESIAN_POINT ( 'NONE',  ( 266.9165763529819628, -52.00000000000000711, 108.9999999999999858 ) ) ;
#45995=ORIENTED_EDGE ( 'NONE', *, *, #11262, .F. ) ;
#45999=EDGE_CURVE ( 'NONE', #16122, #62233, #52314, .T. ) ;
#46010=ORIENTED_EDGE ( 'NONE', *, *, #37497, .T. ) ;
#46043=EDGE_CURVE ( 'NONE', #66949, #65005, #53509, .T. ) ;
#46050=CARTESIAN_POINT ( 'NONE',  ( -2.000000000000000000, 0.000000000000000000, 378.0000000000000000 ) ) ;
#46061=ORIENTED_EDGE ( 'NONE', *, *, #46259, .T. ) ;
#46092=VERTEX_POINT ( 'NONE', #60370 ) ;
#46100=ORIENTED_EDGE ( 'NONE', *, *, #34487, .T. ) ;
#46146=EDGE_CURVE ( 'NONE', #43260, #69361, #54672, .T. ) ;
#46176=DIRECTION ( 'NONE',  ( 0.000000000000000000, 0.000000000000000000, -1.000000000000000000 ) ) ;
#46205=CIRCLE ( 'NONE', #50685, 245.3095347406802489 ) ;
#46207=CARTESIAN_POINT ( 'NONE',  ( 188.9999999999999432, 192.0000000000000000, 72.99999999999998579 ) ) ;
#46216=CIRCLE ( 'NONE', #66484, 5.000000000000004441 ) ;
#46226=DIRECTION ( 'NONE',  ( 0.000000000000000000, 0.02271222823333339177, -0.9997420440737084801 ) ) ;
#46259=EDGE_CURVE ( 'NONE', #2957, #11118, #9248, .T. ) ;
#46274=DIRECTION ( 'NONE',  ( -0.000000000000000000, 0.9989683093773507050, 0.04541273895899262947 ) ) ;
#46286=EDGE_CURVE ( 'NONE', #54192, #5133, #61410, .T. ) ;
#46303=CARTESIAN_POINT ( 'NONE',  ( 259.4165763529819060, 225.8585178651493948, 108.9999999999999858 ) ) ;
#46315=ORIENTED_EDGE ( 'NONE', *, *, #15787, .T. ) ;
#46348=ORIENTED_EDGE ( 'NONE', *, *, #21045, .F. ) ;
#46362=VERTEX_POINT ( 'NONE', #21184 ) ;
#46364=PLANE ( 'NONE',  #64830 ) ;
#46432=ORIENTED_EDGE ( 'NONE', *, *, #57584, .F. ) ;
#46433=EDGE_CURVE ( 'NONE', #51614, #47553, #54558, .T. ) ;
#46464=AXIS2_PLACEMENT_3D ( 'NONE', #55799, #7622, #2338 ) ;
#46484=ORIENTED_EDGE ( 'NONE', *, *, #45038, .T. ) ;
#46486=LINE ( 'NONE', #57395, #7194 ) ;
#46515=ORIENTED_EDGE ( 'NONE', *, *, #48997, .T. ) ;
#46540=DIRECTION ( 'NONE',  ( 0.000000000000000000, 1.000000000000000000, 0.000000000000000000 ) ) ;
#46571=FACE_OUTER_BOUND ( 'NONE', #3221, .T. ) ;
#46579=( NAMED_UNIT ( * ) PLANE_ANGLE_UNIT ( ) SI_UNIT ( $, .RADIAN. ) );
#46590=FACE_OUTER_BOUND ( 'NONE', #6206, .T. ) ;
#46597=CIRCLE ( 'NONE', #55583, 5.000000000000000888 ) ;
#46614=ORIENTED_EDGE ( 'NONE', *, *, #29230, .F. ) ;
#46619=DIRECTION ( 'NONE',  ( 1.000000000000000000, 0.000000000000000000, 0.000000000000000000 ) ) ;
#46651=VECTOR ( 'NONE', #30521, 1000.000000000000000 ) ;
#46653=ORIENTED_EDGE ( 'NONE', *, *, #18122, .T. ) ;
#46711=AXIS2_PLACEMENT_3D ( 'NONE', #22672, #56078, #60656 ) ;
#46763=EDGE_CURVE ( 'NONE', #58078, #53458, #19897, .T. ) ;
#46765=PLANE ( 'NONE',  #38829 ) ;
#46773=DIRECTION ( 'NONE',  ( -0.000000000000000000, 1.000000000000000000, -0.000000000000000000 ) ) ;
#46800=ORIENTED_EDGE ( 'NONE', *, *, #64965, .F. ) ;
#46853=CARTESIAN_POINT ( 'NONE',  ( 209.3223706822284100, 0.000000000000000000, 31.44247402469554942 ) ) ;
#46859=DIRECTION ( 'NONE',  ( -1.000000000000000000, 0.000000000000000000, 0.000000000000000000 ) ) ;
#46881=EDGE_CURVE ( 'NONE', #29599, #5435, #25272, .T. ) ;
#46894=DIRECTION ( 'NONE',  ( 0.000000000000000000, 0.000000000000000000, 1.000000000000000000 ) ) ;
#46938=EDGE_CURVE ( 'NONE', #2243, #41180, #64614, .T. ) ;
#46941=ORIENTED_EDGE ( 'NONE', *, *, #67054, .F. ) ;
#46956=VECTOR ( 'NONE', #45611, 1000.000000000000000 ) ;
#46959=LINE ( 'NONE', #37091, #55967 ) ;
#46963=CARTESIAN_POINT ( 'NONE',  ( 427.4999999999999432, -18.06806526123148160, 378.0000000000000000 ) ) ;
#46985=ORIENTED_EDGE ( 'NONE', *, *, #46881, .F. ) ;
#46999=EDGE_LOOP ( 'NONE', ( #21022, #7765 ) ) ;
#47025=CARTESIAN_POINT ( 'NONE',  ( 209.3223706822284100, 172.0000000000000284, 276.7520087653757628 ) ) ;
#47060=VERTEX_POINT ( 'NONE', #54389 ) ;
#47090=ORIENTED_EDGE ( 'NONE', *, *, #5770, .F. ) ;
#47131=CIRCLE ( 'NONE', #38136, 5.000000000000000888 ) ;
#47133=ORIENTED_EDGE ( 'NONE', *, *, #54366, .T. ) ;
#47152=CARTESIAN_POINT ( 'NONE',  ( 0.000000000000000000, 0.000000000000000000, -2.000000000000000000 ) ) ;
#47155=ORIENTED_EDGE ( 'NONE', *, *, #44236, .T. ) ;
#47211=DIRECTION ( 'NONE',  ( -0.000000000000000000, -0.000000000000000000, -1.000000000000000000 ) ) ;
#47217=CARTESIAN_POINT ( 'NONE',  ( -35.00000000000002842, 225.0000000000000000, -2.000000000000000000 ) ) ;
#47222=FACE_OUTER_BOUND ( 'NONE', #52701, .T. ) ;
#47241=LINE ( 'NONE', #9972, #50997 ) ;
#47268=VECTOR ( 'NONE', #116, 1000.000000000000000 ) ;
#47334=CARTESIAN_POINT ( 'NONE',  ( 111.9975424824652634, 172.0000000000000284, 354.1673509436691347 ) ) ;
#47390=ORIENTED_EDGE ( 'NONE', *, *, #66408, .F. ) ;
#47450=AXIS2_PLACEMENT_3D ( 'NONE', #21086, #10860, #58692 ) ;
#47503=AXIS2_PLACEMENT_3D ( 'NONE', #19568, #24852, #45953 ) ;
#47535=AXIS2_PLACEMENT_3D ( 'NONE', #64109, #37716, #15920 ) ;
#47553=VERTEX_POINT ( 'NONE', #67578 ) ;
#47558=CARTESIAN_POINT ( 'NONE',  ( 264.4165763529819628, 225.8585178651493948, 108.9999999999999858 ) ) ;
#47565=DIRECTION ( 'NONE',  ( 0.000000000000000000, 0.000000000000000000, 1.000000000000000000 ) ) ;
#47575=FACE_OUTER_BOUND ( 'NONE', #50985, .T. ) ;
#47580=CARTESIAN_POINT ( 'NONE',  ( 230.9999999999999432, 190.0000000000000000, -2.000000000000000000 ) ) ;
#47586=CIRCLE ( 'NONE', #50983, 5.000000000000000888 ) ;
#47600=VECTOR ( 'NONE', #29074, 1000.000000000000114 ) ;
#47612=ORIENTED_EDGE ( 'NONE', *, *, #5955, .F. ) ;
#47625=ORIENTED_EDGE ( 'NONE', *, *, #5149, .T. ) ;
#47679=CARTESIAN_POINT ( 'NONE',  ( 309.8720357909272707, 0.000000000000000000, 256.6193948016162381 ) ) ;
#47689=CARTESIAN_POINT ( 'NONE',  ( 311.9975424824652350, 170.0000000000000284, 256.6193948016162381 ) ) ;
#47708=ORIENTED_EDGE ( 'NONE', *, *, #49704, .F. ) ;
#47746=ORIENTED_EDGE ( 'NONE', *, *, #18535, .F. ) ;
#47824=VERTEX_POINT ( 'NONE', #32870 ) ;
#47835=ORIENTED_EDGE ( 'NONE', *, *, #13517, .F. ) ;
#47880=LINE ( 'NONE', #10589, #3933 ) ;
#47894=DIRECTION ( 'NONE',  ( 0.000000000000000000, 0.000000000000000000, 1.000000000000000000 ) ) ;
#47918=FACE_OUTER_BOUND ( 'NONE', #66324, .T. ) ;
#47920=CARTESIAN_POINT ( 'NONE',  ( 109.9975424824652777, 172.0000000000000284, 418.0000000000000000 ) ) ;
#47926=LINE ( 'NONE', #39138, #39992 ) ;
#48079=EDGE_CURVE ( 'NONE', #26166, #7837, #62737, .T. ) ;
#48088=ADVANCED_FACE ( 'NONE', ( #19467 ), #52172, .F. ) ;
#48109=CARTESIAN_POINT ( 'NONE',  ( 188.9999999999999432, -2.000000000000000000, 0.000000000000000000 ) ) ;
#48112=EDGE_LOOP ( 'NONE', ( #15091, #10117, #46315, #69240 ) ) ;
#48115=CARTESIAN_POINT ( 'NONE',  ( 149.4165763529819344, -26.99999999999998224, 129.0000000000000000 ) ) ;
#48118=FACE_BOUND ( 'NONE', #31656, .T. ) ;
#48126=DIRECTION ( 'NONE',  ( -1.000000000000000000, 0.000000000000000000, -0.000000000000000000 ) ) ;
#48135=VECTOR ( 'NONE', #17169, 1000.000000000000000 ) ;
#48144=LINE ( 'NONE', #27042, #41996 ) ;
#48158=ORIENTED_EDGE ( 'NONE', *, *, #41069, .T. ) ;
#48168=LINE ( 'NONE', #53450, #54816 ) ;
#48196=LINE ( 'NONE', #41565, #39397 ) ;
#48240=DIRECTION ( 'NONE',  ( 0.000000000000000000, 0.02271222823333339177, -0.9997420440737084801 ) ) ;
#48258=EDGE_CURVE ( 'NONE', #11698, #65661, #48168, .T. ) ;
#48277=DIRECTION ( 'NONE',  ( 0.000000000000000000, 0.000000000000000000, -1.000000000000000000 ) ) ;
#48302=ORIENTED_EDGE ( 'NONE', *, *, #40114, .T. ) ;
#48308=EDGE_CURVE ( 'NONE', #22151, #58159, #32368, .T. ) ;
#48312=ORIENTED_EDGE ( 'NONE', *, *, #33270, .T. ) ;
#48314=ADVANCED_FACE ( 'NONE', ( #6337 ), #37983, .T. ) ;
#48350=VERTEX_POINT ( 'NONE', #16528 ) ;
#48357=LINE ( 'NONE', #47679, #60711 ) ;
#48395=EDGE_CURVE ( 'NONE', #32729, #23927, #66827, .T. ) ;
#48424=EDGE_CURVE ( 'NONE', #55222, #11778, #34110, .T. ) ;
#48440=PLANE ( 'NONE',  #67686 ) ;
#48443=ORIENTED_EDGE ( 'NONE', *, *, #3813, .F. ) ;
#48451=DIRECTION ( 'NONE',  ( -1.000000000000000000, 0.000000000000000000, 0.000000000000000000 ) ) ;
#48464=CARTESIAN_POINT ( 'NONE',  ( 444.9999999999999432, -35.00000000000000000, 380.0000000000000000 ) ) ;
#48474=CYLINDRICAL_SURFACE ( 'NONE', #34129, 5.000000000000000888 ) ;
#48494=LINE ( 'NONE', #330, #61277 ) ;
#48512=DIRECTION ( 'NONE',  ( 0.000000000000000000, -0.000000000000000000, 1.000000000000000000 ) ) ;
#48582=AXIS2_PLACEMENT_3D ( 'NONE', #10227, #35595, #3574 ) ;
#48590=CARTESIAN_POINT ( 'NONE',  ( 307.2575771313985342, 0.000000000000000000, 256.6193948016162381 ) ) ;
#48633=VECTOR ( 'NONE', #47894, 1000.000000000000000 ) ;
#48638=CARTESIAN_POINT ( 'NONE',  ( 211.9978709542735373, 172.0000000000000284, 276.7363262511108815 ) ) ;
#48677=CYLINDRICAL_SURFACE ( 'NONE', #50079, 5.000000000000004441 ) ;
#48699=CARTESIAN_POINT ( 'NONE',  ( 0.000000000000000000, 192.0000000000000000, 380.0000000000000000 ) ) ;
#48761=DIRECTION ( 'NONE',  ( 0.000000000000000000, 0.000000000000000000, -1.000000000000000000 ) ) ;
#48779=DIRECTION ( 'NONE',  ( -1.000000000000000000, 0.000000000000000000, 0.000000000000000000 ) ) ;
#48801=VERTEX_POINT ( 'NONE', #22766 ) ;
#48837=DIRECTION ( 'NONE',  ( -0.000000000000000000, -0.000000000000000000, -1.000000000000000000 ) ) ;
#48843=ORIENTED_EDGE ( 'NONE', *, *, #33051, .F. ) ;
#48866=DIRECTION ( 'NONE',  ( 0.000000000000000000, 0.9989683093773507050, 0.04541273895899305274 ) ) ;
#48875=ADVANCED_FACE ( 'NONE', ( #47575 ), #56507, .F. ) ;
#48887=EDGE_LOOP ( 'NONE', ( #10132, #38037, #4461, #28586, #23692, #33886, #25160, #477 ) ) ;
#48905=EDGE_CURVE ( 'NONE', #69498, #51848, #21213, .T. ) ;
#48938=CARTESIAN_POINT ( 'NONE',  ( 311.9975424824652350, 20.00000000000003197, 256.6193948016162381 ) ) ;
#48944=CARTESIAN_POINT ( 'NONE',  ( -17.50000000000002842, -18.06806526123148160, 378.0000000000000000 ) ) ;
#48966=ORIENTED_EDGE ( 'NONE', *, *, #28865, .F. ) ;
#48978=DIRECTION ( 'NONE',  ( 0.000000000000000000, 1.000000000000000000, 0.000000000000000000 ) ) ;
#48981=LINE ( 'NONE', #43708, #67359 ) ;
#48986=DIRECTION ( 'NONE',  ( -0.000000000000000000, -0.000000000000000000, -1.000000000000000000 ) ) ;
#48995=DIRECTION ( 'NONE',  ( -0.000000000000000000, -0.000000000000000000, -1.000000000000000000 ) ) ;
#48997=EDGE_CURVE ( 'NONE', #2626, #9719, #22945, .T. ) ;
#49005=ORIENTED_EDGE ( 'NONE', *, *, #44479, .F. ) ;
#49092=AXIS2_PLACEMENT_3D ( 'NONE', #69050, #41988, #19494 ) ;
#49110=CARTESIAN_POINT ( 'NONE',  ( 313.9975424824652350, 172.0000000000000284, 536.6193948016162949 ) ) ;
#49112=DIRECTION ( 'NONE',  ( 1.000000000000000000, -0.000000000000000000, -0.000000000000000000 ) ) ;
#49168=DIRECTION ( 'NONE',  ( -0.000000000000000000, 1.000000000000000000, -0.000000000000000000 ) ) ;
#49170=DIRECTION ( 'NONE',  ( -0.8496664383351307803, 0.000000000000000000, 0.5273205320930463014 ) ) ;
#49217=CARTESIAN_POINT ( 'NONE',  ( 427.4999999999999432, -18.06806526123148160, 380.0000000000000000 ) ) ;
#49230=EDGE_LOOP ( 'NONE', ( #38843, #49848, #31332, #59572 ) ) ;
#49231=CARTESIAN_POINT ( 'NONE',  ( 209.9999999999999716, 0.000000000000000000, 72.99999999999998579 ) ) ;
#49238=ORIENTED_EDGE ( 'NONE', *, *, #59796, .T. ) ;
#49283=ORIENTED_EDGE ( 'NONE', *, *, #46146, .T. ) ;
#49339=ORIENTED_EDGE ( 'NONE', *, *, #1852, .F. ) ;
#49340=ORIENTED_EDGE ( 'NONE', *, *, #14536, .F. ) ;
#49365=EDGE_CURVE ( 'NONE', #69128, #68503, #4264, .T. ) ;
#49379=EDGE_LOOP ( 'NONE', ( #65838, #43730, #62862, #12619 ) ) ;
#49387=DIRECTION ( 'NONE',  ( -0.000000000000000000, -0.000000000000000000, -1.000000000000000000 ) ) ;
#49389=VECTOR ( 'NONE', #53658, 1000.000000000000000 ) ;
#49393=DIRECTION ( 'NONE',  ( 1.000000000000000000, 0.000000000000000000, 0.000000000000000000 ) ) ;
#49415=DIRECTION ( 'NONE',  ( -0.000000000000000000, -0.000000000000000000, -1.000000000000000000 ) ) ;
#49424=EDGE_LOOP ( 'NONE', ( #14919, #49495, #15795, #39008, #61462, #59018 ) ) ;
#49431=PLANE ( 'NONE',  #15885 ) ;
#49441=LINE ( 'NONE', #58961, #63191 ) ;
#49449=ADVANCED_FACE ( 'NONE', ( #14121 ), #35584, .F. ) ;
#49454=ADVANCED_FACE ( 'NONE', ( #1060 ), #10906, .F. ) ;
#49495=ORIENTED_EDGE ( 'NONE', *, *, #68136, .T. ) ;
#49522=DIRECTION ( 'NONE',  ( 1.000000000000000000, -0.000000000000000000, 0.000000000000000000 ) ) ;
#49523=CARTESIAN_POINT ( 'NONE',  ( 209.3223706822284100, 190.0000000000000000, 31.44247402469554942 ) ) ;
#49525=PLANE ( 'NONE',  #37046 ) ;
#49561=VECTOR ( 'NONE', #15600, 1000.000000000000000 ) ;
#49562=DIRECTION ( 'NONE',  ( -1.000000000000000000, 0.000000000000000000, 0.000000000000000000 ) ) ;
#49575=FACE_OUTER_BOUND ( 'NONE', #21242, .T. ) ;
#49579=DIRECTION ( 'NONE',  ( -0.000000000000000000, 1.000000000000000000, 0.000000000000000000 ) ) ;
#49597=EDGE_CURVE ( 'NONE', #60279, #68666, #50986, .T. ) ;
#49605=ADVANCED_FACE ( 'NONE', ( #66147, #49575 ), #44307, .F. ) ;
#49626=VECTOR ( 'NONE', #45022, 1000.000000000000000 ) ;
#49638=DIRECTION ( 'NONE',  ( -0.000000000000000000, -0.000000000000000000, 1.000000000000000000 ) ) ;
#49667=AXIS2_PLACEMENT_3D ( 'NONE', #48115, #42513, #53050 ) ;
#49672=ORIENTED_EDGE ( 'NONE', *, *, #58213, .F. ) ;
#49704=EDGE_CURVE ( 'NONE', #58183, #37385, #31269, .T. ) ;
#49733=LINE ( 'NONE', #18097, #11551 ) ;
#49745=CARTESIAN_POINT ( 'NONE',  ( 410.0000000000000000, 0.000000000000000000, 380.0000000000000000 ) ) ;
#49765=ORIENTED_EDGE ( 'NONE', *, *, #12412, .T. ) ;
#49772=EDGE_CURVE ( 'NONE', #34394, #14640, #9114, .T. ) ;
#49819=VERTEX_POINT ( 'NONE', #32299 ) ;
#49848=ORIENTED_EDGE ( 'NONE', *, *, #58667, .T. ) ;
#49849=ADVANCED_FACE ( 'NONE', ( #43866 ), #27005, .F. ) ;
#49852=VERTEX_POINT ( 'NONE', #11171 ) ;
#49859=VECTOR ( 'NONE', #46619, 1000.000000000000000 ) ;
#49961=CARTESIAN_POINT ( 'NONE',  ( 0.000000000000000000, 190.0000000000000000, 380.0000000000000000 ) ) ;
#49964=AXIS2_PLACEMENT_3D ( 'NONE', #4950, #37643, #21809 ) ;
#49982=ORIENTED_EDGE ( 'NONE', *, *, #4195, .F. ) ;
#49989=CARTESIAN_POINT ( 'NONE',  ( 0.000000000000000000, 0.000000000000000000, -2.000000000000000000 ) ) ;
#49992=FACE_OUTER_BOUND ( 'NONE', #20418, .T. ) ;
#50010=EDGE_CURVE ( 'NONE', #27646, #35609, #22236, .T. ) ;
#50037=DIRECTION ( 'NONE',  ( 1.000000000000000000, 0.000000000000000000, 0.000000000000000000 ) ) ;
#50048=VERTEX_POINT ( 'NONE', #4442 ) ;
#50079=AXIS2_PLACEMENT_3D ( 'NONE', #21969, #11403, #54309 ) ;
#50081=CARTESIAN_POINT ( 'NONE',  ( 209.3223706822284100, 18.00000000000002842, 277.8007638641562380 ) ) ;
#50084=ORIENTED_EDGE ( 'NONE', *, *, #3333, .F. ) ;
#50088=CARTESIAN_POINT ( 'NONE',  ( -35.00000000000002842, 225.0000000000000000, 380.0000000000000000 ) ) ;
#50093=UNCERTAINTY_MEASURE_WITH_UNIT (LENGTH_MEASURE( 1.000000000000000082E-05 ), #61431, 'distance_accuracy_value', 'NONE');
#50121=ORIENTED_EDGE ( 'NONE', *, *, #49704, .T. ) ;
#50149=DIRECTION ( 'NONE',  ( -0.000000000000000000, -0.000000000000000000, 1.000000000000000000 ) ) ;
#50170=FACE_OUTER_BOUND ( 'NONE', #654, .T. ) ;
#50184=CARTESIAN_POINT ( 'NONE',  ( 313.9975424824652350, 18.00000000000002842, 401.6295345748407613 ) ) ;
#50185=ADVANCED_FACE ( 'NONE', ( #25904, #36802 ), #21993, .F. ) ;
#50188=EDGE_CURVE ( 'NONE', #42236, #55222, #40223, .T. ) ;
#50287=LINE ( 'NONE', #55198, #41696 ) ;
#50336=DIRECTION ( 'NONE',  ( 0.000000000000000000, 0.000000000000000000, -1.000000000000000000 ) ) ;
#50407=CYLINDRICAL_SURFACE ( 'NONE', #43275, 5.000000000000004441 ) ;
#50417=EDGE_CURVE ( 'NONE', #16169, #39050, #33449, .T. ) ;
#50421=EDGE_LOOP ( 'NONE', ( #52194, #61683, #45995, #25943 ) ) ;
#50491=ADVANCED_FACE ( 'NONE', ( #46571 ), #67358, .F. ) ;
#50497=ADVANCED_FACE ( 'NONE', ( #67018 ), #36024, .F. ) ;
#50499=LINE ( 'NONE', #59989, #1848 ) ;
#50530=CARTESIAN_POINT ( 'NONE',  ( 0.000000000000000000, 0.000000000000000000, 0.000000000000000000 ) ) ;
#50546=DIRECTION ( 'NONE',  ( 0.000000000000000000, 1.000000000000000000, 0.000000000000000000 ) ) ;
#50547=ORIENTED_EDGE ( 'NONE', *, *, #31980, .T. ) ;
#50576=LINE ( 'NONE', #29817, #8410 ) ;
#50581=ORIENTED_EDGE ( 'NONE', *, *, #40174, .F. ) ;
#50597=DIRECTION ( 'NONE',  ( 0.000000000000000000, 0.000000000000000000, 1.000000000000000000 ) ) ;
#50626=CYLINDRICAL_SURFACE ( 'NONE', #53970, 5.000000000000004441 ) ;
#50640=CARTESIAN_POINT ( 'NONE',  ( 209.9999999999999716, -57.00000000000007816, 72.99999999999998579 ) ) ;
#50645=ORIENTED_EDGE ( 'NONE', *, *, #15956, .T. ) ;
#50651=VERTEX_POINT ( 'NONE', #59709 ) ;
#50668=DIRECTION ( 'NONE',  ( -0.000000000000000000, -0.000000000000000000, -1.000000000000000000 ) ) ;
#50680=EDGE_CURVE ( 'NONE', #58183, #53205, #32993, .T. ) ;
#50684=DIRECTION ( 'NONE',  ( -1.000000000000000000, -0.000000000000000000, -0.000000000000000000 ) ) ;
#50685=AXIS2_PLACEMENT_3D ( 'NONE', #6138, #37810, #60311 ) ;
#50743=DIRECTION ( 'NONE',  ( 2.220446049250313081E-16, -0.000000000000000000, 1.000000000000000000 ) ) ;
#50800=VECTOR ( 'NONE', #56181, 1000.000000000000000 ) ;
#50804=DIRECTION ( 'NONE',  ( 0.000000000000000000, 1.000000000000000000, 0.000000000000000000 ) ) ;
#50841=CARTESIAN_POINT ( 'NONE',  ( 141.9165763529819344, -2.000000000000000000, 108.9999999999999858 ) ) ;
#50850=VECTOR ( 'NONE', #6608, 1000.000000000000000 ) ;
#50851=FACE_OUTER_BOUND ( 'NONE', #57303, .T. ) ;
#50857=DIRECTION ( 'NONE',  ( 0.000000000000000000, 0.000000000000000000, -1.000000000000000000 ) ) ;
#50864=DIRECTION ( 'NONE',  ( 1.000000000000000000, 0.000000000000000000, 0.000000000000000000 ) ) ;
#50867=DIRECTION ( 'NONE',  ( 0.000000000000000000, 1.000000000000000000, 0.000000000000000000 ) ) ;
#50932=ORIENTED_EDGE ( 'NONE', *, *, #37724, .F. ) ;
#50952=DIRECTION ( 'NONE',  ( -0.000000000000000000, -1.000000000000000000, -0.000000000000000000 ) ) ;
#50964=CARTESIAN_POINT ( 'NONE',  ( 444.9999999999999432, -35.00000000000000000, 380.0000000000000000 ) ) ;
#50983=AXIS2_PLACEMENT_3D ( 'NONE', #54847, #60828, #49562 ) ;
#50985=EDGE_LOOP ( 'NONE', ( #21936, #19647, #58082, #8695 ) ) ;
#50986=LINE ( 'NONE', #2115, #32291 ) ;
#50991=EDGE_CURVE ( 'NONE', #37589, #14950, #44063, .T. ) ;
#50997=VECTOR ( 'NONE', #31423, 1000.000000000000000 ) ;
#51006=CARTESIAN_POINT ( 'NONE',  ( 109.9975424824652634, 179.2896996249788799, 369.5505932007772003 ) ) ;
#51008=CARTESIAN_POINT ( 'NONE',  ( 444.9999999999999432, -35.00000000000000000, 0.000000000000000000 ) ) ;
#51031=ORIENTED_EDGE ( 'NONE', *, *, #49597, .T. ) ;
#51042=VECTOR ( 'NONE', #51320, 1000.000000000000000 ) ;
#51064=ADVANCED_FACE ( 'NONE', ( #59201 ), #16643, .F. ) ;
#51071=ADVANCED_FACE ( 'NONE', ( #16984 ), #826, .F. ) ;
#51091=EDGE_CURVE ( 'NONE', #45635, #5291, #27543, .T. ) ;
#51132=CIRCLE ( 'NONE', #39926, 21.00000000000000355 ) ;
#51154=VECTOR ( 'NONE', #30679, 1000.000000000000000 ) ;
#51161=CYLINDRICAL_SURFACE ( 'NONE', #23422, 5.000000000000004441 ) ;
#51167=EDGE_LOOP ( 'NONE', ( #68638, #5326, #38186, #30110 ) ) ;
#51181=EDGE_CURVE ( 'NONE', #24965, #11879, #2909, .T. ) ;
#51194=DIRECTION ( 'NONE',  ( 0.000000000000000000, -0.000000000000000000, 1.000000000000000000 ) ) ;
#51195=CARTESIAN_POINT ( 'NONE',  ( 188.9999999999999432, 225.0000000000000000, -2.000000000000000888 ) ) ;
#51213=VERTEX_POINT ( 'NONE', #67626 ) ;
#51233=EDGE_CURVE ( 'NONE', #21755, #16701, #24892, .T. ) ;
#51249=CARTESIAN_POINT ( 'NONE',  ( 209.9999999999999716, -57.00000000000007816, 72.99999999999998579 ) ) ;
#51254=CIRCLE ( 'NONE', #37720, 246.3582898394606957 ) ;
#51291=ADVANCED_FACE ( 'NONE', ( #40880 ), #62341, .F. ) ;
#51320=DIRECTION ( 'NONE',  ( 0.000000000000000000, 0.000000000000000000, -1.000000000000000000 ) ) ;
#51337=VECTOR ( 'NONE', #42124, 1000.000000000000000 ) ;
#51345=CARTESIAN_POINT ( 'NONE',  ( -22.50000000000003197, 207.5000000000000284, -2.000000000000000000 ) ) ;
#51426=AXIS2_PLACEMENT_3D ( 'NONE', #9289, #8258, #29711 ) ;
#51442=CARTESIAN_POINT ( 'NONE',  ( 427.4999999999999432, 207.5000000000000284, 378.0000000000000000 ) ) ;
#51445=DIRECTION ( 'NONE',  ( -0.000000000000000000, 1.000000000000000000, -0.000000000000000000 ) ) ;
#51449=CARTESIAN_POINT ( 'NONE',  ( 410.9216045519012823, 190.0000000000000000, 173.9247703311572764 ) ) ;
#51469=DIRECTION ( 'NONE',  ( -0.000000000000000000, -0.000000000000000000, -1.000000000000000000 ) ) ;
#51471=CARTESIAN_POINT ( 'NONE',  ( 266.9165763529819628, 242.0000000000000000, 128.9999999999999716 ) ) ;
#51487=ADVANCED_FACE ( 'NONE', ( #11624 ), #32744, .F. ) ;
#51513=DIRECTION ( 'NONE',  ( -1.000000000000000000, 0.000000000000000000, 0.000000000000000000 ) ) ;
#51558=CARTESIAN_POINT ( 'NONE',  ( 422.4999999999999432, 207.5000000000000284, 380.0000000000000000 ) ) ;
#51614=VERTEX_POINT ( 'NONE', #9144 ) ;
#51653=EDGE_CURVE ( 'NONE', #51213, #35609, #35534, .T. ) ;
#51661=EDGE_LOOP ( 'NONE', ( #3403, #25437, #44486, #9735 ) ) ;
#51677=LINE ( 'NONE', #62584, #56001 ) ;
#51706=EDGE_CURVE ( 'NONE', #48801, #34756, #46216, .T. ) ;
#51711=ADVANCED_FACE ( 'NONE', ( #38544 ), #49431, .T. ) ;
#51730=AXIS2_PLACEMENT_3D ( 'NONE', #15265, #48277, #69053 ) ;
#51739=LINE ( 'NONE', #24672, #26568 ) ;
#51760=VECTOR ( 'NONE', #28017, 1000.000000000000000 ) ;
#51762=ADVANCED_FACE ( 'NONE', ( #22717 ), #1974, .F. ) ;
#51774=EDGE_LOOP ( 'NONE', ( #1464, #48966, #61703, #42399 ) ) ;
#51802=CARTESIAN_POINT ( 'NONE',  ( 410.0000000000000000, 0.000000000000000000, 175.2157797990580832 ) ) ;
#51816=DIRECTION ( 'NONE',  ( 0.000000000000000000, 0.000000000000000000, 1.000000000000000000 ) ) ;
#51817=EDGE_LOOP ( 'NONE', ( #61550, #59589, #58390, #11194 ) ) ;
#51818=ORIENTED_EDGE ( 'NONE', *, *, #54648, .T. ) ;
#51841=AXIS2_PLACEMENT_3D ( 'NONE', #26072, #10570, #26417 ) ;
#51848=VERTEX_POINT ( 'NONE', #50841 ) ;
#51850=PLANE ( 'NONE',  #10800 ) ;
#51853=CARTESIAN_POINT ( 'NONE',  ( 427.4999999999999432, -18.06806526123148160, 378.0000000000000000 ) ) ;
#51854=FACE_BOUND ( 'NONE', #66856, .T. ) ;
#51857=AXIS2_PLACEMENT_3D ( 'NONE', #8210, #46176, #24045 ) ;
#51875=LINE ( 'NONE', #40978, #10739 ) ;
#51901=CIRCLE ( 'NONE', #5838, 245.3095347406802489 ) ;
#51941=AXIS2_PLACEMENT_3D ( 'NONE', #32668, #657, #17167 ) ;
#51949=ADVANCED_FACE ( 'NONE', ( #5062 ), #57849, .F. ) ;
#51964=ORIENTED_EDGE ( 'NONE', *, *, #30989, .T. ) ;
#51966=LINE ( 'NONE', #56552, #21467 ) ;
#51978=EDGE_LOOP ( 'NONE', ( #7118, #65192, #69317, #45119 ) ) ;
#51985=LINE ( 'NONE', #68511, #45068 ) ;
#52022=DIRECTION ( 'NONE',  ( 0.000000000000000000, 0.000000000000000000, 1.000000000000000000 ) ) ;
#52047=DIRECTION ( 'NONE',  ( 0.000000000000000000, 0.000000000000000000, 1.000000000000000000 ) ) ;
#52055=DIRECTION ( 'NONE',  ( 2.220446049250313081E-16, 0.000000000000000000, 1.000000000000000000 ) ) ;
#52074=EDGE_LOOP ( 'NONE', ( #59799, #66898 ) ) ;
#52086=ORIENTED_EDGE ( 'NONE', *, *, #14382, .F. ) ;
#52088=ORIENTED_EDGE ( 'NONE', *, *, #12416, .F. ) ;
#52112=ORIENTED_EDGE ( 'NONE', *, *, #21051, .F. ) ;
#52115=ORIENTED_EDGE ( 'NONE', *, *, #60502, .T. ) ;
#52172=PLANE ( 'NONE',  #33509 ) ;
#52187=CYLINDRICAL_SURFACE ( 'NONE', #36869, 5.000000000000000888 ) ;
#52194=ORIENTED_EDGE ( 'NONE', *, *, #356, .F. ) ;
#52209=FILL_AREA_STYLE ('',( #53223 ) ) ;
#52215=ORIENTED_EDGE ( 'NONE', *, *, #50188, .T. ) ;
#52220=PLANE ( 'NONE',  #18805 ) ;
#52231=VECTOR ( 'NONE', #5246, 1000.000000000000000 ) ;
#52238=CARTESIAN_POINT ( 'NONE',  ( 109.9975424824652634, 172.0000000000000284, 418.0000000000000568 ) ) ;
#52239=DIRECTION ( 'NONE',  ( -1.000000000000000000, 0.000000000000000000, 0.000000000000000000 ) ) ;
#52265=CARTESIAN_POINT ( 'NONE',  ( 311.9975424824652350, 170.0000000000000284, 256.6193948016162381 ) ) ;
#52282=AXIS2_PLACEMENT_3D ( 'NONE', #14939, #68742, #10689 ) ;
#52295=LINE ( 'NONE', #47689, #58292 ) ;
#52314=LINE ( 'NONE', #41766, #8606 ) ;
#52338=VERTEX_POINT ( 'NONE', #30614 ) ;
#52350=VECTOR ( 'NONE', #40546, 1000.000000000000000 ) ;
#52352=VERTEX_POINT ( 'NONE', #69268 ) ;
#52358=DIRECTION ( 'NONE',  ( -1.000000000000000000, 0.000000000000000000, 0.000000000000000000 ) ) ;
#52374=ORIENTED_EDGE ( 'NONE', *, *, #21208, .F. ) ;
#52375=AXIS2_PLACEMENT_3D ( 'NONE', #27553, #48995, #37413 ) ;
#52379=VECTOR ( 'NONE', #35213, 1000.000000000000000 ) ;
#52442=FACE_BOUND ( 'NONE', #33838, .T. ) ;
#52443=EDGE_CURVE ( 'NONE', #57527, #11698, #29409, .T. ) ;
#52456=VERTEX_POINT ( 'NONE', #54453 ) ;
#52472=CARTESIAN_POINT ( 'NONE',  ( 209.3223706822284100, 0.000000000000000000, 31.44247402469554942 ) ) ;
#52540=CARTESIAN_POINT ( 'NONE',  ( 0.000000000000000000, 190.0000000000000000, 380.0000000000000000 ) ) ;
#52566=VECTOR ( 'NONE', #4665, 1000.000000000000000 ) ;
#52577=FACE_OUTER_BOUND ( 'NONE', #24366, .T. ) ;
#52629=EDGE_LOOP ( 'NONE', ( #45657, #53020, #22175, #58271 ) ) ;
#52664=CARTESIAN_POINT ( 'NONE',  ( 213.7144841804914392, 190.0000000000000000, 277.7626788299629652 ) ) ;
#52701=EDGE_LOOP ( 'NONE', ( #2902, #30410, #36110, #67537 ) ) ;
#52744=CARTESIAN_POINT ( 'NONE',  ( 444.9999999999999432, 225.0000000000000000, -2.000000000000000000 ) ) ;
#52752=ORIENTED_EDGE ( 'NONE', *, *, #56079, .T. ) ;
#52823=CARTESIAN_POINT ( 'NONE',  ( 141.9165763529819344, -2.000000000000001776, 129.0000000000000000 ) ) ;
#52861=EDGE_CURVE ( 'NONE', #62679, #18878, #69366, .T. ) ;
#52870=ORIENTED_EDGE ( 'NONE', *, *, #46259, .F. ) ;
#52883=PRESENTATION_STYLE_ASSIGNMENT (( #63112 ) ) ;
#52892=AXIS2_PLACEMENT_3D ( 'NONE', #3602, #3953, #46859 ) ;
#52914=ORIENTED_EDGE ( 'NONE', *, *, #43171, .T. ) ;
#52932=EDGE_CURVE ( 'NONE', #50048, #2626, #44044, .T. ) ;
#52948=EDGE_CURVE ( 'NONE', #54192, #29393, #24998, .T. ) ;
#52954=DIRECTION ( 'NONE',  ( 0.000000000000000000, -0.000000000000000000, -1.000000000000000000 ) ) ;
#52980=LINE ( 'NONE', #4803, #28033 ) ;
#52989=CARTESIAN_POINT ( 'NONE',  ( 444.9999999999999432, -35.00000000000000000, 380.0000000000000000 ) ) ;
#53020=ORIENTED_EDGE ( 'NONE', *, *, #57584, .T. ) ;
#53050=DIRECTION ( 'NONE',  ( 1.000000000000000000, 0.000000000000000000, 0.000000000000000000 ) ) ;
#53087=CARTESIAN_POINT ( 'NONE',  ( 149.4165763529819344, -26.99999999999998224, 138.9999999999999716 ) ) ;
#53161=ORIENTED_EDGE ( 'NONE', *, *, #63925, .F. ) ;
#53170=CARTESIAN_POINT ( 'NONE',  ( 410.0000000000000000, 0.000000000000000000, -2.000000000000000000 ) ) ;
#53172=ORIENTED_EDGE ( 'NONE', *, *, #10644, .T. ) ;
#53179=DIRECTION ( 'NONE',  ( -0.000000000000000000, -0.000000000000000000, -1.000000000000000000 ) ) ;
#53205=VERTEX_POINT ( 'NONE', #16081 ) ;
#53207=VECTOR ( 'NONE', #13089, 1000.000000000000000 ) ;
#53208=CARTESIAN_POINT ( 'NONE',  ( 266.9165763529819628, -52.00000000000000711, 128.9999999999999716 ) ) ;
#53210=CARTESIAN_POINT ( 'NONE',  ( 109.9975424824652634, 18.00000000000002842, 401.6295345748407613 ) ) ;
#53220=AXIS2_PLACEMENT_3D ( 'NONE', #41433, #15388, #36154 ) ;
#53223=FILL_AREA_STYLE_COLOUR ( '', #6490 ) ;
#53241=DIRECTION ( 'NONE',  ( -1.000000000000000000, 0.000000000000000000, 0.000000000000000000 ) ) ;
#53274=VECTOR ( 'NONE', #38663, 1000.000000000000000 ) ;
#53308=AXIS2_PLACEMENT_3D ( 'NONE', #5554, #64300, #33607 ) ;
#53341=ORIENTED_EDGE ( 'NONE', *, *, #61209, .F. ) ;
#53385=ORIENTED_EDGE ( 'NONE', *, *, #69390, .F. ) ;
#53398=EDGE_CURVE ( 'NONE', #66949, #69361, #12912, .T. ) ;
#53401=EDGE_CURVE ( 'NONE', #57196, #30930, #34368, .T. ) ;
#53406=ORIENTED_EDGE ( 'NONE', *, *, #57399, .F. ) ;
#53409=FACE_OUTER_BOUND ( 'NONE', #52629, .T. ) ;
#53416=CARTESIAN_POINT ( 'NONE',  ( -35.00000000000002842, 225.0000000000000000, 380.0000000000000000 ) ) ;
#53450=CARTESIAN_POINT ( 'NONE',  ( -12.50000000000002842, 207.5000000000000284, 378.0000000000000000 ) ) ;
#53458=VERTEX_POINT ( 'NONE', #43843 ) ;
#53459=ORIENTED_EDGE ( 'NONE', *, *, #27290, .F. ) ;
#53474=ORIENTED_EDGE ( 'NONE', *, *, #14554, .F. ) ;
#53497=DIRECTION ( 'NONE',  ( -0.000000000000000000, -1.000000000000000000, 0.000000000000000000 ) ) ;
#53500=CARTESIAN_POINT ( 'NONE',  ( 307.2575771313985342, 0.000000000000000000, 256.6193948016162381 ) ) ;
#53509=CIRCLE ( 'NONE', #23218, 5.000000000000004441 ) ;
#53512=CARTESIAN_POINT ( 'NONE',  ( 313.9975424824652350, 172.0000000000000284, 256.6193948016162381 ) ) ;
#53516=AXIS2_PLACEMENT_3D ( 'NONE', #68603, #15492, #10193 ) ;
#53527=FACE_OUTER_BOUND ( 'NONE', #36462, .T. ) ;
#53530=VECTOR ( 'NONE', #6649, 1000.000000000000000 ) ;
#53556=AXIS2_PLACEMENT_3D ( 'NONE', #27718, #58710, #10185 ) ;
#53560=DIRECTION ( 'NONE',  ( 0.000000000000000000, -1.000000000000000000, 0.000000000000000000 ) ) ;
#53563=CARTESIAN_POINT ( 'NONE',  ( 111.9975424824652634, 179.2896996249788799, 369.5505932007772003 ) ) ;
#53576=CARTESIAN_POINT ( 'NONE',  ( -12.50000000000002842, -18.06806526123148160, 0.000000000000000000 ) ) ;
#53597=DIRECTION ( 'NONE',  ( 0.000000000000000000, 1.000000000000000000, 0.000000000000000000 ) ) ;
#53630=SHAPE_DEFINITION_REPRESENTATION ( #14271, #57739 ) ;
#53638=DIRECTION ( 'NONE',  ( -0.000000000000000000, -1.000000000000000000, -0.000000000000000000 ) ) ;
#53646=CARTESIAN_POINT ( 'NONE',  ( 111.9975424824652634, 170.0000000000000284, 256.6193948016162381 ) ) ;
#53658=DIRECTION ( 'NONE',  ( 0.000000000000000000, 1.000000000000000000, -0.000000000000000000 ) ) ;
#53682=DIRECTION ( 'NONE',  ( 0.000000000000000000, 0.000000000000000000, -1.000000000000000000 ) ) ;
#53729=DIRECTION ( 'NONE',  ( 0.000000000000000000, -1.000000000000000000, 0.000000000000000000 ) ) ;
#53735=CARTESIAN_POINT ( 'NONE',  ( 141.9165763529819344, 242.0000000000000000, 129.0000000000000000 ) ) ;
#53755=ORIENTED_EDGE ( 'NONE', *, *, #62591, .T. ) ;
#53760=DIRECTION ( 'NONE',  ( -0.000000000000000000, -1.000000000000000000, -0.000000000000000000 ) ) ;
#53767=DIRECTION ( 'NONE',  ( 1.000000000000000000, 0.000000000000000000, 0.000000000000000000 ) ) ;
#53781=EDGE_LOOP ( 'NONE', ( #33812, #61308 ) ) ;
#53800=FACE_BOUND ( 'NONE', #9386, .T. ) ;
#53806=FACE_OUTER_BOUND ( 'NONE', #49424, .T. ) ;
#53833=DIRECTION ( 'NONE',  ( -0.000000000000000000, 1.000000000000000000, -0.000000000000000000 ) ) ;
#53854=AXIS2_PLACEMENT_3D ( 'NONE', #27191, #6083, #11711 ) ;
#53866=CARTESIAN_POINT ( 'NONE',  ( 211.9978709542735373, 18.00000000000003553, 276.7363262511108815 ) ) ;
#53891=AXIS2_PLACEMENT_3D ( 'NONE', #46963, #31148, #67738 ) ;
#53903=EDGE_CURVE ( 'NONE', #54103, #68068, #65503, .T. ) ;
#53931=CARTESIAN_POINT ( 'NONE',  ( -12.50000000000002842, 207.5000000000000284, 0.000000000000000000 ) ) ;
#53932=ORIENTED_EDGE ( 'NONE', *, *, #24472, .F. ) ;
#53943=ORIENTED_EDGE ( 'NONE', *, *, #66738, .T. ) ;
#53944=ORIENTED_EDGE ( 'NONE', *, *, #62591, .F. ) ;
#53970=AXIS2_PLACEMENT_3D ( 'NONE', #55917, #55205, #66836 ) ;
#53974=ORIENTED_EDGE ( 'NONE', *, *, #46433, .F. ) ;
#53988=CARTESIAN_POINT ( 'NONE',  ( 313.9975424824652350, 18.08738615523480675, 402.4289050101931480 ) ) ;
#54024=VECTOR ( 'NONE', #6255, 1000.000000000000000 ) ;
#54074=VECTOR ( 'NONE', #34922, 1000.000000000000114 ) ;
#54083=DIRECTION ( 'NONE',  ( 0.000000000000000000, 0.000000000000000000, -1.000000000000000000 ) ) ;
#54091=ORIENTED_EDGE ( 'NONE', *, *, #39362, .F. ) ;
#54103=VERTEX_POINT ( 'NONE', #42485 ) ;
#54124=CARTESIAN_POINT ( 'NONE',  ( 109.9975424824652777, 172.0000000000000284, 418.0000000000000000 ) ) ;
#54151=EDGE_CURVE ( 'NONE', #16482, #9638, #15753, .T. ) ;
#54172=DIRECTION ( 'NONE',  ( 2.220446049250313081E-16, -0.000000000000000000, 1.000000000000000000 ) ) ;
#54174=CARTESIAN_POINT ( 'NONE',  ( 444.9999999999999432, -35.00000000000000000, -2.000000000000000000 ) ) ;
#54192=VERTEX_POINT ( 'NONE', #42815 ) ;
#54213=EDGE_CURVE ( 'NONE', #55507, #14375, #39640, .T. ) ;
#54262=VECTOR ( 'NONE', #51469, 1000.000000000000000 ) ;
#54289=DIRECTION ( 'NONE',  ( -0.000000000000000000, -1.000000000000000000, -0.000000000000000000 ) ) ;
#54309=DIRECTION ( 'NONE',  ( -1.000000000000000000, 0.000000000000000000, 0.000000000000000000 ) ) ;
#54359=AXIS2_PLACEMENT_3D ( 'NONE', #44942, #13296, #3425 ) ;
#54366=EDGE_CURVE ( 'NONE', #65444, #454, #6228, .T. ) ;
#54387=FACE_OUTER_BOUND ( 'NONE', #180, .T. ) ;
#54389=CARTESIAN_POINT ( 'NONE',  ( 254.4165763529819344, 225.8585178651493948, 128.9999999999999716 ) ) ;
#54430=CARTESIAN_POINT ( 'NONE',  ( 141.9165763529819344, -52.00000000000000711, 129.0000000000000000 ) ) ;
#54452=CARTESIAN_POINT ( 'NONE',  ( 0.000000000000000000, 0.000000000000000000, 161.3522585083728700 ) ) ;
#54453=CARTESIAN_POINT ( 'NONE',  ( 213.7147529443549843, 18.00000000000002132, 277.7621479143228385 ) ) ;
#54463=VECTOR ( 'NONE', #49168, 1000.000000000000000 ) ;
#54467=EDGE_CURVE ( 'NONE', #40644, #9181, #8222, .T. ) ;
#54498=EDGE_LOOP ( 'NONE', ( #59704, #8871, #59502, #41029 ) ) ;
#54504=ORIENTED_EDGE ( 'NONE', *, *, #28078, .F. ) ;
#54507=ORIENTED_EDGE ( 'NONE', *, *, #59468, .F. ) ;
#54534=ORIENTED_EDGE ( 'NONE', *, *, #36949, .F. ) ;
#54537=ORIENTED_EDGE ( 'NONE', *, *, #27376, .F. ) ;
#54558=LINE ( 'NONE', #27840, #60308 ) ;
#54610=DIRECTION ( 'NONE',  ( 0.000000000000000000, 0.000000000000000000, -1.000000000000000000 ) ) ;
#54618=FACE_OUTER_BOUND ( 'NONE', #39713, .T. ) ;
#54619=ADVANCED_FACE ( 'NONE', ( #6140 ), #43768, .T. ) ;
#54621=CARTESIAN_POINT ( 'NONE',  ( 311.9975424824652350, 20.00000000000003197, 380.0000000000001137 ) ) ;
#54646=DIRECTION ( 'NONE',  ( -1.000000000000000000, 0.000000000000000000, 0.000000000000000000 ) ) ;
#54648=EDGE_CURVE ( 'NONE', #20901, #66152, #13181, .T. ) ;
#54653=ORIENTED_EDGE ( 'NONE', *, *, #58572, .F. ) ;
#54672=CIRCLE ( 'NONE', #62523, 5.000000000000004441 ) ;
#54692=PLANE ( 'NONE',  #33565 ) ;
#54728=LINE ( 'NONE', #39267, #56508 ) ;
#54748=CARTESIAN_POINT ( 'NONE',  ( 0.000000000000000000, 192.0000000000000000, 378.0000000000000000 ) ) ;
#54755=VERTEX_POINT ( 'NONE', #69396 ) ;
#54759=DIRECTION ( 'NONE',  ( -0.000000000000000000, 1.000000000000000000, -0.000000000000000000 ) ) ;
#54778=EDGE_CURVE ( 'NONE', #50048, #21528, #47241, .T. ) ;
#54783=EDGE_LOOP ( 'NONE', ( #10849, #4647, #45244, #19084 ) ) ;
#54784=DIRECTION ( 'NONE',  ( 1.000000000000000000, 0.000000000000000000, -0.000000000000000000 ) ) ;
#54811=FACE_OUTER_BOUND ( 'NONE', #62509, .T. ) ;
#54816=VECTOR ( 'NONE', #42897, 1000.000000000000000 ) ;
#54847=CARTESIAN_POINT ( 'NONE',  ( -17.50000000000002842, -18.06806526123148160, -2.000000000000000000 ) ) ;
#54905=DIRECTION ( 'NONE',  ( -1.000000000000000000, 0.000000000000000000, 0.000000000000000000 ) ) ;
#54935=EDGE_CURVE ( 'NONE', #29393, #26090, #33515, .T. ) ;
#54940=CARTESIAN_POINT ( 'NONE',  ( 154.4165763529819628, -26.99999999999998224, 138.9999999999999716 ) ) ;
#54977=ORIENTED_EDGE ( 'NONE', *, *, #48424, .F. ) ;
#55025=CARTESIAN_POINT ( 'NONE',  ( 0.000000000000000000, 0.000000000000000000, 380.0000000000000000 ) ) ;
#55045=FACE_OUTER_BOUND ( 'NONE', #65247, .T. ) ;
#55050=ADVANCED_BREP_SHAPE_REPRESENTATION ( '', ( #62812, #66832 ), #11761 ) ;
#55074=LINE ( 'NONE', #28351, #11002 ) ;
#55084=ORIENTED_EDGE ( 'NONE', *, *, #11642, .T. ) ;
#55156=FACE_OUTER_BOUND ( 'NONE', #59435, .T. ) ;
#55182=ORIENTED_EDGE ( 'NONE', *, *, #15413, .F. ) ;
#55198=CARTESIAN_POINT ( 'NONE',  ( 188.9999999999999432, -2.000000000000000000, 380.0000000000000000 ) ) ;
#55205=DIRECTION ( 'NONE',  ( -0.000000000000000000, -0.000000000000000000, 1.000000000000000000 ) ) ;
#55206=VECTOR ( 'NONE', #38131, 1000.000000000000000 ) ;
#55217=ORIENTED_EDGE ( 'NONE', *, *, #39925, .T. ) ;
#55219=FACE_OUTER_BOUND ( 'NONE', #17205, .T. ) ;
#55222=VERTEX_POINT ( 'NONE', #37995 ) ;
#55228=LINE ( 'NONE', #24288, #42489 ) ;
#55236=LINE ( 'NONE', #38022, #29900 ) ;
#55258=VERTEX_POINT ( 'NONE', #42908 ) ;
#55301=AXIS2_PLACEMENT_3D ( 'NONE', #63631, #4874, #57663 ) ;
#55340=DIRECTION ( 'NONE',  ( -1.000000000000000000, 0.000000000000000000, 0.000000000000000000 ) ) ;
#55344=CARTESIAN_POINT ( 'NONE',  ( 311.9975424824652350, -23.68493792952219934, 521.0102483033961107 ) ) ;
#55377=FACE_OUTER_BOUND ( 'NONE', #51661, .T. ) ;
#55391=CIRCLE ( 'NONE', #59847, 160.5210298272983778 ) ;
#55397=CIRCLE ( 'NONE', #43030, 245.3095347406803342 ) ;
#55412=CARTESIAN_POINT ( 'NONE',  ( 209.3223706822284100, 172.0000000000000284, 31.44247402469554942 ) ) ;
#55425=CARTESIAN_POINT ( 'NONE',  ( 0.000000000000000000, 0.000000000000000000, 380.0000000000000000 ) ) ;
#55444=VECTOR ( 'NONE', #2251, 1000.000000000000114 ) ;
#55450=DIRECTION ( 'NONE',  ( -0.000000000000000000, -0.000000000000000000, -1.000000000000000000 ) ) ;
#55457=AXIS2_PLACEMENT_3D ( 'NONE', #55025, #49393, #527 ) ;
#55470=LINE ( 'NONE', #17486, #37470 ) ;
#55486=EDGE_CURVE ( 'NONE', #33294, #37589, #17047, .T. ) ;
#55492=DIRECTION ( 'NONE',  ( 0.000000000000000000, 1.000000000000000000, -0.000000000000000000 ) ) ;
#55507=VERTEX_POINT ( 'NONE', #67014 ) ;
#55534=CARTESIAN_POINT ( 'NONE',  ( -35.00000000000002842, -35.00000000000000000, 0.000000000000000000 ) ) ;
#55535=PLANE ( 'NONE',  #44292 ) ;
#55548=DIRECTION ( 'NONE',  ( 0.000000000000000000, 0.000000000000000000, 1.000000000000000000 ) ) ;
#55555=FACE_OUTER_BOUND ( 'NONE', #4514, .T. ) ;
#55571=VERTEX_POINT ( 'NONE', #24781 ) ;
#55572=DIRECTION ( 'NONE',  ( 0.000000000000000000, 0.000000000000000000, 1.000000000000000000 ) ) ;
#55580=DIRECTION ( 'NONE',  ( 1.000000000000000000, -0.000000000000000000, -0.000000000000000000 ) ) ;
#55583=AXIS2_PLACEMENT_3D ( 'NONE', #31808, #26187, #53241 ) ;
#55636=VECTOR ( 'NONE', #27809, 1000.000000000000000 ) ;
#55650=AXIS2_PLACEMENT_3D ( 'NONE', #41323, #4032, #25503 ) ;
#55678=CARTESIAN_POINT ( 'NONE',  ( 313.9975424824652350, 170.0000000000000284, 536.6193948016162949 ) ) ;
#55705=DIRECTION ( 'NONE',  ( 1.000000000000000000, -0.000000000000000000, -0.000000000000000000 ) ) ;
#55710=EDGE_LOOP ( 'NONE', ( #63491, #57684, #31824, #23358 ) ) ;
#55721=DIRECTION ( 'NONE',  ( -0.000000000000000000, -0.000000000000000000, -1.000000000000000000 ) ) ;
#55735=DIRECTION ( 'NONE',  ( -0.000000000000000000, -1.000000000000000000, -0.000000000000000000 ) ) ;
#55739=CARTESIAN_POINT ( 'NONE',  ( 412.0000000000000000, 0.000000000000000000, 378.0000000000000000 ) ) ;
#55743=EDGE_CURVE ( 'NONE', #53205, #63094, #31775, .T. ) ;
#55762=EDGE_LOOP ( 'NONE', ( #35782, #20371, #25218, #45009, #57758, #17501, #61103, #67254 ) ) ;
#55799=CARTESIAN_POINT ( 'NONE',  ( 262.2186286510350328, 0.000000000000000000, 236.5504542314483274 ) ) ;
#55828=CARTESIAN_POINT ( 'NONE',  ( 213.7150814747576817, 0.000000000000000000, 277.7615984639418798 ) ) ;
#55840=FACE_OUTER_BOUND ( 'NONE', #35594, .T. ) ;
#55844=VERTEX_POINT ( 'NONE', #6431 ) ;
#55917=CARTESIAN_POINT ( 'NONE',  ( 427.4999999999999432, -18.06806526123148160, 378.0000000000000000 ) ) ;
#55936=DIRECTION ( 'NONE',  ( 1.000000000000000000, 0.000000000000000000, -0.000000000000000000 ) ) ;
#55955=ORIENTED_EDGE ( 'NONE', *, *, #23656, .T. ) ;
#55956=DIRECTION ( 'NONE',  ( -0.000000000000000000, -0.000000000000000000, -1.000000000000000000 ) ) ;
#55967=VECTOR ( 'NONE', #25174, 1000.000000000000000 ) ;
#55979=ORIENTED_EDGE ( 'NONE', *, *, #65946, .T. ) ;
#56001=VECTOR ( 'NONE', #14398, 1000.000000000000000 ) ;
#56011=DIRECTION ( 'NONE',  ( -1.000000000000000000, 0.000000000000000000, 0.000000000000000000 ) ) ;
#56063=DIRECTION ( 'NONE',  ( -0.000000000000000000, 1.000000000000000000, -0.000000000000000000 ) ) ;
#56074=FACE_OUTER_BOUND ( 'NONE', #57963, .T. ) ;
#56078=DIRECTION ( 'NONE',  ( 0.000000000000000000, 1.000000000000000000, 0.000000000000000000 ) ) ;
#56079=EDGE_CURVE ( 'NONE', #28546, #4522, #44642, .T. ) ;
#56096=ORIENTED_EDGE ( 'NONE', *, *, #39086, .F. ) ;
#56097=DIRECTION ( 'NONE',  ( 0.000000000000000000, 0.000000000000000000, 1.000000000000000000 ) ) ;
#56098=AXIS2_PLACEMENT_3D ( 'NONE', #52540, #53560, #57826 ) ;
#56114=CARTESIAN_POINT ( 'NONE',  ( 0.000000000000000000, 242.0000000000000000, 0.000000000000000000 ) ) ;
#56142=CARTESIAN_POINT ( 'NONE',  ( 309.8720357909272707, 170.0000000000000284, 256.6193948016162381 ) ) ;
#56148=( NAMED_UNIT ( * ) PLANE_ANGLE_UNIT ( ) SI_UNIT ( $, .RADIAN. ) );
#56163=CARTESIAN_POINT ( 'NONE',  ( 188.9999999999999432, 190.0000000000000000, -2.000000000000000888 ) ) ;
#56176=VECTOR ( 'NONE', #55705, 1000.000000000000000 ) ;
#56181=DIRECTION ( 'NONE',  ( -1.000000000000000000, -0.000000000000000000, -0.000000000000000000 ) ) ;
#56207=DIRECTION ( 'NONE',  ( 0.000000000000000000, 0.000000000000000000, -1.000000000000000000 ) ) ;
#56211=DIRECTION ( 'NONE',  ( -0.000000000000000000, 1.000000000000000000, -0.000000000000000000 ) ) ;
#56217=DIRECTION ( 'NONE',  ( 0.000000000000000000, 1.000000000000000000, 0.000000000000000000 ) ) ;
#56224=EDGE_CURVE ( 'NONE', #10473, #49852, #35075, .T. ) ;
#56246=ORIENTED_EDGE ( 'NONE', *, *, #14382, .T. ) ;
#56285=VERTEX_POINT ( 'NONE', #8701 ) ;
#56302=ORIENTED_EDGE ( 'NONE', *, *, #21499, .F. ) ;
#56312=DIRECTION ( 'NONE',  ( -1.000000000000000000, 0.000000000000000000, 0.000000000000000000 ) ) ;
#56318=VECTOR ( 'NONE', #19343, 1000.000000000000000 ) ;
#56339=DIRECTION ( 'NONE',  ( -0.000000000000000000, -0.000000000000000000, -1.000000000000000000 ) ) ;
#56396=DIRECTION ( 'NONE',  ( -1.000000000000000000, 0.000000000000000000, 0.000000000000000000 ) ) ;
#56402=DIRECTION ( 'NONE',  ( -0.000000000000000000, -0.000000000000000000, -1.000000000000000000 ) ) ;
#56442=EDGE_CURVE ( 'NONE', #53458, #23927, #31527, .T. ) ;
#56454=VERTEX_POINT ( 'NONE', #37836 ) ;
#56456=FACE_OUTER_BOUND ( 'NONE', #35480, .T. ) ;
#56470=EDGE_CURVE ( 'NONE', #29725, #20901, #37572, .T. ) ;
#56507=CYLINDRICAL_SURFACE ( 'NONE', #13321, 21.00000000000000355 ) ;
#56508=VECTOR ( 'NONE', #65652, 1000.000000000000000 ) ;
#56550=EDGE_LOOP ( 'NONE', ( #18829, #48443, #46061, #33025 ) ) ;
#56552=CARTESIAN_POINT ( 'NONE',  ( 188.9999999999999432, -0.000000000000000000, 0.000000000000000000 ) ) ;
#56570=CYLINDRICAL_SURFACE ( 'NONE', #31854, 245.3095347406802205 ) ;
#56577=DIRECTION ( 'NONE',  ( -1.000000000000000000, 0.000000000000000000, 0.000000000000000000 ) ) ;
#56620=ORIENTED_EDGE ( 'NONE', *, *, #21499, .T. ) ;
#56653=VERTEX_POINT ( 'NONE', #68055 ) ;
#56659=LINE ( 'NONE', #68262, #40144 ) ;
#56695=EDGE_CURVE ( 'NONE', #29393, #14950, #18473, .T. ) ;
#56737=PLANE ( 'NONE',  #1717 ) ;
#56749=DIRECTION ( 'NONE',  ( 0.000000000000000000, 0.000000000000000000, -1.000000000000000000 ) ) ;
#56757=LINE ( 'NONE', #8579, #60318 ) ;
#56778=DIRECTION ( 'NONE',  ( 0.000000000000000000, 0.000000000000000000, -1.000000000000000000 ) ) ;
#56796=CARTESIAN_POINT ( 'NONE',  ( 311.9975424824652350, 20.00000000000003197, 256.6193948016162381 ) ) ;
#56800=CARTESIAN_POINT ( 'NONE',  ( 109.9975424824652634, 296.0000000000000000, 529.9060149868646477 ) ) ;
#56831=ORIENTED_EDGE ( 'NONE', *, *, #44105, .T. ) ;
#56898=CARTESIAN_POINT ( 'NONE',  ( 109.9975424824652634, 20.00000000000003197, 536.6193948016162949 ) ) ;
#56900=ORIENTED_EDGE ( 'NONE', *, *, #38759, .T. ) ;
#56902=ADVANCED_FACE ( 'NONE', ( #21914 ), #59537, .T. ) ;
#56930=CARTESIAN_POINT ( 'NONE',  ( 313.9975424824652350, 296.0000000000000000, 418.0000000000000000 ) ) ;
#56960=EDGE_CURVE ( 'NONE', #21528, #9719, #62335, .T. ) ;
#56967=CARTESIAN_POINT ( 'NONE',  ( 311.9975424824652350, 20.00000000000003197, 254.5114349394235091 ) ) ;
#57042=CARTESIAN_POINT ( 'NONE',  ( 111.9975424824652634, 295.8720703627916464, 535.5371946177799600 ) ) ;
#57063=VECTOR ( 'NONE', #20200, 1000.000000000000000 ) ;
#57118=CARTESIAN_POINT ( 'NONE',  ( 444.9999999999999432, 225.0000000000000000, -2.000000000000000000 ) ) ;
#57128=EDGE_CURVE ( 'NONE', #13740, #22362, #992, .T. ) ;
#57141=DIRECTION ( 'NONE',  ( -0.000000000000000000, -0.000000000000000000, -1.000000000000000000 ) ) ;
#57176=CARTESIAN_POINT ( 'NONE',  ( 432.4999999999999432, -18.06806526123148160, 0.000000000000000000 ) ) ;
#57180=ORIENTED_EDGE ( 'NONE', *, *, #41691, .F. ) ;
#57196=VERTEX_POINT ( 'NONE', #2047 ) ;
#57214=ORIENTED_EDGE ( 'NONE', *, *, #38759, .F. ) ;
#57264=VERTEX_POINT ( 'NONE', #24548 ) ;
#57277=DIRECTION ( 'NONE',  ( 0.000000000000000000, 1.000000000000000000, -0.000000000000000000 ) ) ;
#57284=FACE_OUTER_BOUND ( 'NONE', #23894, .T. ) ;
#57303=EDGE_LOOP ( 'NONE', ( #29710, #40029, #27738, #17924, #63527, #2048, #65083 ) ) ;
#57308=CARTESIAN_POINT ( 'NONE',  ( 264.4165763529819628, -27.00000000000000355, 108.9999999999999858 ) ) ;
#57330=CARTESIAN_POINT ( 'NONE',  ( 209.3223706822284100, 0.000000000000000000, 277.8007638641562380 ) ) ;
#57379=DIRECTION ( 'NONE',  ( -0.000000000000000000, -0.000000000000000000, -1.000000000000000000 ) ) ;
#57395=CARTESIAN_POINT ( 'NONE',  ( 311.9975424824652350, 172.0000000000000284, 527.9060149868646477 ) ) ;
#57399=EDGE_CURVE ( 'NONE', #14754, #34394, #27633, .T. ) ;
#57430=LINE ( 'NONE', #55425, #54262 ) ;
#57443=ORIENTED_EDGE ( 'NONE', *, *, #44466, .F. ) ;
#57444=ORIENTED_EDGE ( 'NONE', *, *, #39192, .F. ) ;
#57450=ORIENTED_EDGE ( 'NONE', *, *, #50991, .F. ) ;
#57467=FACE_BOUND ( 'NONE', #26676, .T. ) ;
#57493=LINE ( 'NONE', #20888, #57063 ) ;
#57522=VECTOR ( 'NONE', #67204, 1000.000000000000000 ) ;
#57527=VERTEX_POINT ( 'NONE', #45905 ) ;
#57528=ORIENTED_EDGE ( 'NONE', *, *, #61409, .T. ) ;
#57584=EDGE_CURVE ( 'NONE', #22014, #66758, #57917, .T. ) ;
#57606=ADVANCED_FACE ( 'NONE', ( #37404 ), #57841, .F. ) ;
#57618=CARTESIAN_POINT ( 'NONE',  ( 266.9165763529819628, 242.0000000000000000, 108.9999999999999858 ) ) ;
#57641=LINE ( 'NONE', #15416, #2035 ) ;
#57655=DIRECTION ( 'NONE',  ( 1.000000000000000000, 0.000000000000000000, 0.000000000000000000 ) ) ;
#57663=DIRECTION ( 'NONE',  ( 0.000000000000000000, 0.000000000000000000, -1.000000000000000000 ) ) ;
#57675=FACE_OUTER_BOUND ( 'NONE', #51774, .T. ) ;
#57684=ORIENTED_EDGE ( 'NONE', *, *, #62279, .F. ) ;
#57707=ORIENTED_EDGE ( 'NONE', *, *, #23599, .T. ) ;
#57714=VERTEX_POINT ( 'NONE', #4381 ) ;
#57739=SHAPE_REPRESENTATION ( 'Part1', ( #66832 ), #11761 ) ;
#57746=ORIENTED_EDGE ( 'NONE', *, *, #34004, .F. ) ;
#57754=CARTESIAN_POINT ( 'NONE',  ( 444.9999999999999432, 225.0000000000000000, 380.0000000000000000 ) ) ;
#57758=ORIENTED_EDGE ( 'NONE', *, *, #52948, .F. ) ;
#57777=LINE ( 'NONE', #52823, #48633 ) ;
#57787=ORIENTED_EDGE ( 'NONE', *, *, #11103, .F. ) ;
#57821=ORIENTED_EDGE ( 'NONE', *, *, #58160, .T. ) ;
#57825=DIRECTION ( 'NONE',  ( 0.000000000000000000, -0.000000000000000000, 1.000000000000000000 ) ) ;
#57826=DIRECTION ( 'NONE',  ( 0.000000000000000000, -0.000000000000000000, -1.000000000000000000 ) ) ;
#57829=PLANE ( 'NONE',  #49092 ) ;
#57841=PLANE ( 'NONE',  #29856 ) ;
#57849=PLANE ( 'NONE',  #4690 ) ;
#57853=AXIS2_PLACEMENT_3D ( 'NONE', #33200, #64509, #42700 ) ;
#57864=ADVANCED_FACE ( 'NONE', ( #64845 ), #50407, .F. ) ;
#57917=CIRCLE ( 'NONE', #55650, 246.3582898394606957 ) ;
#57918=ORIENTED_EDGE ( 'NONE', *, *, #43316, .F. ) ;
#57939=DIRECTION ( 'NONE',  ( -0.000000000000000000, -1.000000000000000000, -0.000000000000000000 ) ) ;
#57963=EDGE_LOOP ( 'NONE', ( #28548, #16385, #18884, #35637 ) ) ;
#57969=AXIS2_PLACEMENT_3D ( 'NONE', #36990, #53833, #68320 ) ;
#57978=ADVANCED_FACE ( 'NONE', ( #34236 ), #1885, .T. ) ;
#57992=DIRECTION ( 'NONE',  ( 0.000000000000000000, 0.000000000000000000, -1.000000000000000000 ) ) ;
#57997=EDGE_CURVE ( 'NONE', #11610, #27523, #40882, .T. ) ;
#58069=ORIENTED_EDGE ( 'NONE', *, *, #52443, .F. ) ;
#58078=VERTEX_POINT ( 'NONE', #29292 ) ;
#58082=ORIENTED_EDGE ( 'NONE', *, *, #15240, .T. ) ;
#58115=ORIENTED_EDGE ( 'NONE', *, *, #40365, .T. ) ;
#58134=ADVANCED_FACE ( 'NONE', ( #42606 ), #37318, .T. ) ;
#58153=CARTESIAN_POINT ( 'NONE',  ( -17.50000000000002842, 207.5000000000000284, -2.000000000000000000 ) ) ;
#58159=VERTEX_POINT ( 'NONE', #41573 ) ;
#58160=EDGE_CURVE ( 'NONE', #68068, #5133, #18654, .T. ) ;
#58170=FACE_BOUND ( 'NONE', #17164, .T. ) ;
#58176=ORIENTED_EDGE ( 'NONE', *, *, #54467, .F. ) ;
#58183=VERTEX_POINT ( 'NONE', #42937 ) ;
#58213=EDGE_CURVE ( 'NONE', #13740, #34313, #51254, .T. ) ;
#58244=DIRECTION ( 'NONE',  ( -1.000000000000000000, 0.000000000000000000, 0.000000000000000000 ) ) ;
#58245=LINE ( 'NONE', #39146, #44082 ) ;
#58271=ORIENTED_EDGE ( 'NONE', *, *, #68136, .F. ) ;
#58274=CARTESIAN_POINT ( 'NONE',  ( 427.4999999999999432, -18.06806526123148160, 0.000000000000000000 ) ) ;
#58283=CARTESIAN_POINT ( 'NONE',  ( 313.9975424824652350, 295.6904194069557548, 539.5330678552892323 ) ) ;
#58292=VECTOR ( 'NONE', #20283, 1000.000000000000000 ) ;
#58293=DIRECTION ( 'NONE',  ( -0.000000000000000000, -1.000000000000000000, -0.000000000000000000 ) ) ;
#58347=DIRECTION ( 'NONE',  ( 0.000000000000000000, 1.000000000000000000, 0.000000000000000000 ) ) ;
#58353=EDGE_CURVE ( 'NONE', #19781, #5206, #55236, .T. ) ;
#58364=DIRECTION ( 'NONE',  ( 1.000000000000000000, 0.000000000000000000, 0.000000000000000000 ) ) ;
#58377=EDGE_LOOP ( 'NONE', ( #11132, #57746 ) ) ;
#58390=ORIENTED_EDGE ( 'NONE', *, *, #69004, .F. ) ;
#58411=PLANE ( 'NONE',  #48582 ) ;
#58438=CARTESIAN_POINT ( 'NONE',  ( -22.50000000000003197, 207.5000000000000284, 380.0000000000000000 ) ) ;
#58448=EDGE_LOOP ( 'NONE', ( #34485, #10521, #12308, #15992 ) ) ;
#58465=DIRECTION ( 'NONE',  ( -1.000000000000000000, 0.000000000000000000, 0.000000000000000000 ) ) ;
#58476=CARTESIAN_POINT ( 'NONE',  ( -22.50000000000003197, -18.06806526123148160, 378.0000000000000000 ) ) ;
#58481=LINE ( 'NONE', #42661, #59042 ) ;
#58501=VECTOR ( 'NONE', #45266, 1000.000000000000000 ) ;
#58511=EDGE_CURVE ( 'NONE', #61576, #57714, #3869, .T. ) ;
#58528=ORIENTED_EDGE ( 'NONE', *, *, #12947, .T. ) ;
#58542=CARTESIAN_POINT ( 'NONE',  ( -12.50000000000002842, -18.06806526123148160, 378.0000000000000000 ) ) ;
#58544=VECTOR ( 'NONE', #10377, 1000.000000000000000 ) ;
#58572=EDGE_CURVE ( 'NONE', #27491, #536, #61230, .T. ) ;
#58578=DIRECTION ( 'NONE',  ( -0.000000000000000000, -0.000000000000000000, -1.000000000000000000 ) ) ;
#58579=FACE_BOUND ( 'NONE', #58377, .T. ) ;
#58583=DIRECTION ( 'NONE',  ( -0.8532989592251508659, 0.000000000000000000, 0.5214219847544543374 ) ) ;
#58609=ORIENTED_EDGE ( 'NONE', *, *, #61209, .T. ) ;
#58624=ORIENTED_EDGE ( 'NONE', *, *, #40174, .T. ) ;
#58667=EDGE_CURVE ( 'NONE', #26166, #68068, #50499, .T. ) ;
#58675=EDGE_CURVE ( 'NONE', #8163, #29725, #23770, .T. ) ;
#58692=DIRECTION ( 'NONE',  ( 0.000000000000000000, 0.000000000000000000, 1.000000000000000000 ) ) ;
#58697=DIRECTION ( 'NONE',  ( 0.000000000000000000, 0.000000000000000000, -1.000000000000000000 ) ) ;
#58702=DIRECTION ( 'NONE',  ( -0.000000000000000000, -0.000000000000000000, 1.000000000000000000 ) ) ;
#58703=ORIENTED_EDGE ( 'NONE', *, *, #49365, .F. ) ;
#58710=DIRECTION ( 'NONE',  ( 1.000000000000000000, 0.000000000000000000, 0.000000000000000000 ) ) ;
#58726=EDGE_LOOP ( 'NONE', ( #48158, #16306, #54534, #50645, #57443, #49765 ) ) ;
#58728=VERTEX_POINT ( 'NONE', #12877 ) ;
#58736=ORIENTED_EDGE ( 'NONE', *, *, #18931, .T. ) ;
#58793=VECTOR ( 'NONE', #9427, 1000.000000000000000 ) ;
#58838=EDGE_LOOP ( 'NONE', ( #23788, #1399, #21341, #61366, #36902, #39603 ) ) ;
#58844=ORIENTED_EDGE ( 'NONE', *, *, #68920, .T. ) ;
#58875=ORIENTED_EDGE ( 'NONE', *, *, #39245, .T. ) ;
#58888=CIRCLE ( 'NONE', #54359, 245.3095347406802205 ) ;
#58907=VECTOR ( 'NONE', #63881, 1000.000000000000114 ) ;
#58922=ORIENTED_EDGE ( 'NONE', *, *, #20705, .F. ) ;
#58926=FACE_OUTER_BOUND ( 'NONE', #34539, .T. ) ;
#58950=VECTOR ( 'NONE', #58984, 1000.000000000000000 ) ;
#58951=AXIS2_PLACEMENT_3D ( 'NONE', #3500, #24968, #3853 ) ;
#58961=CARTESIAN_POINT ( 'NONE',  ( 111.9975424824652634, 0.000000000000000000, 256.6193948016162381 ) ) ;
#58984=DIRECTION ( 'NONE',  ( 1.000000000000000000, 0.000000000000000000, 0.000000000000000000 ) ) ;
#59018=ORIENTED_EDGE ( 'NONE', *, *, #7336, .T. ) ;
#59037=AXIS2_PLACEMENT_3D ( 'NONE', #8560, #35641, #14177 ) ;
#59041=CIRCLE ( 'NONE', #46711, 246.3582898394606957 ) ;
#59042=VECTOR ( 'NONE', #59173, 1000.000000000000000 ) ;
#59082=PLANE ( 'NONE',  #34083 ) ;
#59137=ORIENTED_EDGE ( 'NONE', *, *, #22332, .T. ) ;
#59159=ORIENTED_EDGE ( 'NONE', *, *, #44236, .F. ) ;
#59171=CARTESIAN_POINT ( 'NONE',  ( 311.9975424824652350, 20.00000000000003197, 401.6295345748407613 ) ) ;
#59173=DIRECTION ( 'NONE',  ( 0.000000000000000000, 1.000000000000000000, 0.000000000000000000 ) ) ;
#59201=FACE_OUTER_BOUND ( 'NONE', #55762, .T. ) ;
#59204=ORIENTED_EDGE ( 'NONE', *, *, #27059, .F. ) ;
#59232=ORIENTED_EDGE ( 'NONE', *, *, #3498, .T. ) ;
#59269=FACE_OUTER_BOUND ( 'NONE', #5499, .T. ) ;
#59274=CARTESIAN_POINT ( 'NONE',  ( 109.9975424824652634, 0.000000000000000000, 256.8908838121927261 ) ) ;
#59278=AXIS2_PLACEMENT_3D ( 'NONE', #60049, #34395, #28047 ) ;
#59301=AXIS2_PLACEMENT_3D ( 'NONE', #66702, #40634, #24485 ) ;
#59312=DIRECTION ( 'NONE',  ( 0.000000000000000000, 0.000000000000000000, -1.000000000000000000 ) ) ;
#59313=ADVANCED_FACE ( 'NONE', ( #54387 ), #37182, .T. ) ;
#59318=DIRECTION ( 'NONE',  ( -0.000000000000000000, -0.000000000000000000, 1.000000000000000000 ) ) ;
#59331=ORIENTED_EDGE ( 'NONE', *, *, #33196, .F. ) ;
#59364=CARTESIAN_POINT ( 'NONE',  ( 311.9975424824652350, 20.00000000000003197, 256.6193948016162381 ) ) ;
#59388=CYLINDRICAL_SURFACE ( 'NONE', #47450, 246.3582898394606957 ) ;
#59432=CARTESIAN_POINT ( 'NONE',  ( 313.9975424824652350, 296.0000000000000000, 529.9060149868646477 ) ) ;
#59435=EDGE_LOOP ( 'NONE', ( #50932, #58922, #57707, #33656 ) ) ;
#59443=EDGE_CURVE ( 'NONE', #18390, #37473, #3375, .T. ) ;
#59468=EDGE_CURVE ( 'NONE', #61512, #25612, #36074, .T. ) ;
#59483=VERTEX_POINT ( 'NONE', #53866 ) ;
#59495=ORIENTED_EDGE ( 'NONE', *, *, #51181, .F. ) ;
#59502=ORIENTED_EDGE ( 'NONE', *, *, #23702, .F. ) ;
#59517=VECTOR ( 'NONE', #54289, 1000.000000000000000 ) ;
#59537=PLANE ( 'NONE',  #44400 ) ;
#59542=ADVANCED_FACE ( 'NONE', ( #53527 ), #22925, .F. ) ;
#59545=DIRECTION ( 'NONE',  ( 0.000000000000000000, 0.000000000000000000, -1.000000000000000000 ) ) ;
#59568=CARTESIAN_POINT ( 'NONE',  ( 444.9999999999999432, -35.00000000000000000, 0.000000000000000000 ) ) ;
#59570=VERTEX_POINT ( 'NONE', #10620 ) ;
#59572=ORIENTED_EDGE ( 'NONE', *, *, #30840, .T. ) ;
#59581=EDGE_CURVE ( 'NONE', #28668, #11879, #20797, .T. ) ;
#59589=ORIENTED_EDGE ( 'NONE', *, *, #21372, .F. ) ;
#59599=ORIENTED_EDGE ( 'NONE', *, *, #26678, .T. ) ;
#59629=ADVANCED_FACE ( 'NONE', ( #61930 ), #61602, .F. ) ;
#59642=ORIENTED_EDGE ( 'NONE', *, *, #23377, .F. ) ;
#59665=CIRCLE ( 'NONE', #51857, 5.000000000000004441 ) ;
#59704=ORIENTED_EDGE ( 'NONE', *, *, #21196, .F. ) ;
#59709=CARTESIAN_POINT ( 'NONE',  ( 213.7144242967635535, -1.188791048788683712E-16, 277.7626972944978547 ) ) ;
#59717=LINE ( 'NONE', #43192, #8110 ) ;
#59718=ORIENTED_EDGE ( 'NONE', *, *, #62824, .F. ) ;
#59731=DIRECTION ( 'NONE',  ( -0.000000000000000000, -0.000000000000000000, -1.000000000000000000 ) ) ;
#59738=DIRECTION ( 'NONE',  ( -2.398676446365434695E-14, 0.000000000000000000, 1.000000000000000000 ) ) ;
#59756=CARTESIAN_POINT ( 'NONE',  ( 410.0000000000000000, 190.0000000000000000, -2.000000000000000000 ) ) ;
#59785=EDGE_CURVE ( 'NONE', #14375, #14640, #37267, .T. ) ;
#59796=EDGE_CURVE ( 'NONE', #2243, #9949, #48494, .T. ) ;
#59799=ORIENTED_EDGE ( 'NONE', *, *, #19864, .F. ) ;
#59804=LINE ( 'NONE', #66171, #55636 ) ;
#59809=VERTEX_POINT ( 'NONE', #59756 ) ;
#59847=AXIS2_PLACEMENT_3D ( 'NONE', #7782, #3202, #30276 ) ;
#59853=AXIS2_PLACEMENT_3D ( 'NONE', #52989, #26277, #63905 ) ;
#59883=LINE ( 'NONE', #11702, #67314 ) ;
#59931=EDGE_CURVE ( 'NONE', #47060, #9181, #14710, .T. ) ;
#59954=ORIENTED_EDGE ( 'NONE', *, *, #57128, .T. ) ;
#59986=LINE ( 'NONE', #41838, #26471 ) ;
#59987=CARTESIAN_POINT ( 'NONE',  ( 309.8720357909272707, 18.00000000000002842, 536.6193948016162949 ) ) ;
#59989=CARTESIAN_POINT ( 'NONE',  ( 311.9975424824652350, 20.00000000000003197, 256.6193948016162381 ) ) ;
#59994=ORIENTED_EDGE ( 'NONE', *, *, #31787, .F. ) ;
#60029=CARTESIAN_POINT ( 'NONE',  ( 410.0000000000000000, 0.000000000000000000, 380.0000000000000000 ) ) ;
#60047=CARTESIAN_POINT ( 'NONE',  ( -12.50000000000002842, 207.5000000000000284, 0.000000000000000000 ) ) ;
#60048=ORIENTED_EDGE ( 'NONE', *, *, #23752, .F. ) ;
#60049=CARTESIAN_POINT ( 'NONE',  ( 427.4999999999999432, 207.5000000000000284, 380.0000000000000000 ) ) ;
#60071=EDGE_CURVE ( 'NONE', #37589, #5460, #29089, .T. ) ;
#60115=AXIS2_PLACEMENT_3D ( 'NONE', #9732, #27268, #58583 ) ;
#60136=ORIENTED_EDGE ( 'NONE', *, *, #15956, .F. ) ;
#60158=ORIENTED_EDGE ( 'NONE', *, *, #55486, .F. ) ;
#60166=DIRECTION ( 'NONE',  ( -1.000000000000000000, 0.000000000000000000, 0.000000000000000000 ) ) ;
#60224=AXIS2_PLACEMENT_3D ( 'NONE', #55678, #7509, #59545 ) ;
#60258=DIRECTION ( 'NONE',  ( -0.000000000000000000, -0.000000000000000000, -1.000000000000000000 ) ) ;
#60279=VERTEX_POINT ( 'NONE', #6133 ) ;
#60308=VECTOR ( 'NONE', #50684, 1000.000000000000000 ) ;
#60311=DIRECTION ( 'NONE',  ( -0.8532989592251507549, 0.000000000000000000, 0.5214219847544545594 ) ) ;
#60318=VECTOR ( 'NONE', #56063, 1000.000000000000000 ) ;
#60325=CARTESIAN_POINT ( 'NONE',  ( 311.9975424824652350, 20.00000000000003197, 401.6295345748407613 ) ) ;
#60326=LINE ( 'NONE', #43781, #38054 ) ;
#60351=DIRECTION ( 'NONE',  ( -1.000000000000000000, 0.000000000000000000, 0.000000000000000000 ) ) ;
#60362=ADVANCED_FACE ( 'NONE', ( #27243 ), #48677, .F. ) ;
#60363=AXIS2_PLACEMENT_3D ( 'NONE', #13844, #46540, #46894 ) ;
#60367=LINE ( 'NONE', #37863, #4253 ) ;
#60368=FACE_OUTER_BOUND ( 'NONE', #38102, .T. ) ;
#60369=VECTOR ( 'NONE', #1595, 1000.000000000000000 ) ;
#60370=CARTESIAN_POINT ( 'NONE',  ( 311.9975424824652350, 170.0000000000000284, 256.6193948016162381 ) ) ;
#60395=DIRECTION ( 'NONE',  ( -0.000000000000000000, 1.000000000000000000, -0.000000000000000000 ) ) ;
#60423=VERTEX_POINT ( 'NONE', #44478 ) ;
#60459=DIRECTION ( 'NONE',  ( 0.000000000000000000, 1.000000000000000000, 0.000000000000000000 ) ) ;
#60481=ORIENTED_EDGE ( 'NONE', *, *, #5871, .T. ) ;
#60489=EDGE_CURVE ( 'NONE', #34313, #50651, #59041, .T. ) ;
#60492=ORIENTED_EDGE ( 'NONE', *, *, #45473, .T. ) ;
#60494=DIRECTION ( 'NONE',  ( 0.000000000000000000, 1.000000000000000000, -0.000000000000000000 ) ) ;
#60502=EDGE_CURVE ( 'NONE', #42281, #60658, #66973, .T. ) ;
#60566=FACE_OUTER_BOUND ( 'NONE', #44955, .T. ) ;
#60605=VECTOR ( 'NONE', #36648, 1000.000000000000000 ) ;
#60645=AXIS2_PLACEMENT_3D ( 'NONE', #40038, #59731, #16829 ) ;
#60647=ORIENTED_EDGE ( 'NONE', *, *, #11103, .T. ) ;
#60656=DIRECTION ( 'NONE',  ( -0.8496664383351307803, 0.000000000000000000, 0.5273205320930463014 ) ) ;
#60658=VERTEX_POINT ( 'NONE', #58476 ) ;
#60694=ORIENTED_EDGE ( 'NONE', *, *, #37368, .T. ) ;
#60711=VECTOR ( 'NONE', #10398, 1000.000000000000000 ) ;
#60739=ORIENTED_EDGE ( 'NONE', *, *, #45473, .F. ) ;
#60759=LINE ( 'NONE', #66756, #44945 ) ;
#60783=CIRCLE ( 'NONE', #52892, 5.000000000000004441 ) ;
#60804=CARTESIAN_POINT ( 'NONE',  ( 422.4999999999999432, -18.06806526123148160, 380.0000000000000000 ) ) ;
#60828=DIRECTION ( 'NONE',  ( 0.000000000000000000, 0.000000000000000000, -1.000000000000000000 ) ) ;
#60871=VECTOR ( 'NONE', #37929, 1000.000000000000000 ) ;
#60920=CIRCLE ( 'NONE', #24989, 245.3095347406802773 ) ;
#60931=ORIENTED_EDGE ( 'NONE', *, *, #3813, .T. ) ;
#60953=DIRECTION ( 'NONE',  ( -1.000000000000000000, 0.000000000000000000, 0.000000000000000000 ) ) ;
#60985=EDGE_CURVE ( 'NONE', #66758, #22108, #39301, .T. ) ;
#61003=DIRECTION ( 'NONE',  ( -0.000000000000000000, -0.000000000000000000, -1.000000000000000000 ) ) ;
#61043=AXIS2_PLACEMENT_3D ( 'NONE', #25094, #30364, #51816 ) ;
#61057=CARTESIAN_POINT ( 'NONE',  ( 311.9975424824652350, 296.0000000000000000, 420.0000000000000000 ) ) ;
#61070=DIRECTION ( 'NONE',  ( -2.692596297684568294E-16, -1.000000000000000000, 1.133976529980832822E-16 ) ) ;
#61071=AXIS2_PLACEMENT_3D ( 'NONE', #431, #5368, #16606 ) ;
#61103=ORIENTED_EDGE ( 'NONE', *, *, #58160, .F. ) ;
#61116=DIRECTION ( 'NONE',  ( 0.000000000000000000, -1.000000000000000000, -0.000000000000000000 ) ) ;
#61137=VECTOR ( 'NONE', #67520, 1000.000000000000000 ) ;
#61143=DIRECTION ( 'NONE',  ( -0.000000000000000000, -0.000000000000000000, -1.000000000000000000 ) ) ;
#61202=LINE ( 'NONE', #22870, #9309 ) ;
#61209=EDGE_CURVE ( 'NONE', #28546, #16482, #44485, .T. ) ;
#61230=CIRCLE ( 'NONE', #32003, 5.000000000000004441 ) ;
#61233=CARTESIAN_POINT ( 'NONE',  ( 211.9972138934681425, 190.0000000000000000, 276.7374251518728556 ) ) ;
#61261=LINE ( 'NONE', #44737, #22931 ) ;
#61266=DIRECTION ( 'NONE',  ( 0.000000000000000000, 0.000000000000000000, -1.000000000000000000 ) ) ;
#61277=VECTOR ( 'NONE', #21115, 1000.000000000000000 ) ;
#61308=ORIENTED_EDGE ( 'NONE', *, *, #18891, .T. ) ;
#61363=ORIENTED_EDGE ( 'NONE', *, *, #49597, .F. ) ;
#61365=EDGE_CURVE ( 'NONE', #52338, #8192, #18796, .T. ) ;
#61366=ORIENTED_EDGE ( 'NONE', *, *, #28054, .T. ) ;
#61409=EDGE_CURVE ( 'NONE', #20810, #37937, #3313, .T. ) ;
#61410=LINE ( 'NONE', #37016, #9748 ) ;
#61431=( LENGTH_UNIT ( ) NAMED_UNIT ( * ) SI_UNIT ( .MILLI., .METRE. ) );
#61442=ORIENTED_EDGE ( 'NONE', *, *, #68240, .T. ) ;
#61462=ORIENTED_EDGE ( 'NONE', *, *, #11176, .T. ) ;
#61474=AXIS2_PLACEMENT_3D ( 'NONE', #48938, #47565, #77 ) ;
#61491=DIRECTION ( 'NONE',  ( 0.000000000000000000, -0.1086713087885527451, -0.9940777367219241212 ) ) ;
#61506=CARTESIAN_POINT ( 'NONE',  ( 209.3223706822284100, 172.0000000000000284, 277.8007638641562380 ) ) ;
#61512=VERTEX_POINT ( 'NONE', #20179 ) ;
#61519=FACE_OUTER_BOUND ( 'NONE', #3979, .T. ) ;
#61537=CIRCLE ( 'NONE', #28956, 5.000000000000004441 ) ;
#61540=VERTEX_POINT ( 'NONE', #26837 ) ;
#61545=CARTESIAN_POINT ( 'NONE',  ( -12.50000000000002842, -18.06806526123148160, -2.000000000000000000 ) ) ;
#61549=DIRECTION ( 'NONE',  ( 0.000000000000000000, 0.000000000000000000, 1.000000000000000000 ) ) ;
#61550=ORIENTED_EDGE ( 'NONE', *, *, #46433, .T. ) ;
#61562=AXIS2_PLACEMENT_3D ( 'NONE', #15345, #58578, #58244 ) ;
#61567=DIRECTION ( 'NONE',  ( -1.000000000000000000, 0.000000000000000000, 0.000000000000000000 ) ) ;
#61576=VERTEX_POINT ( 'NONE', #47580 ) ;
#61602=PLANE ( 'NONE',  #62384 ) ;
#61616=VECTOR ( 'NONE', #15591, 1000.000000000000000 ) ;
#61629=ORIENTED_EDGE ( 'NONE', *, *, #13376, .T. ) ;
#61683=ORIENTED_EDGE ( 'NONE', *, *, #50680, .F. ) ;
#61702=DIRECTION ( 'NONE',  ( 0.000000000000000000, -1.000000000000000000, 0.000000000000000000 ) ) ;
#61703=ORIENTED_EDGE ( 'NONE', *, *, #59796, .F. ) ;
#61721=ORIENTED_EDGE ( 'NONE', *, *, #463, .F. ) ;
#61735=DIRECTION ( 'NONE',  ( 0.000000000000000000, 0.000000000000000000, 1.000000000000000000 ) ) ;
#61739=VERTEX_POINT ( 'NONE', #39140 ) ;
#61772=EDGE_LOOP ( 'NONE', ( #10045, #28781, #18108, #38562 ) ) ;
#61847=CARTESIAN_POINT ( 'NONE',  ( 311.9975424824652350, 172.0000000000000284, 536.6193948016162949 ) ) ;
#61906=DIRECTION ( 'NONE',  ( 0.000000000000000000, 1.000000000000000000, -0.000000000000000000 ) ) ;
#61930=FACE_OUTER_BOUND ( 'NONE', #32656, .T. ) ;
#61931=LINE ( 'NONE', #13755, #52379 ) ;
#61970=VECTOR ( 'NONE', #33849, 1000.000000000000000 ) ;
#61992=CARTESIAN_POINT ( 'NONE',  ( 259.4165763529819060, -27.00000000000000355, 128.9999999999999716 ) ) ;
#62028=FACE_OUTER_BOUND ( 'NONE', #51978, .T. ) ;
#62048=CARTESIAN_POINT ( 'NONE',  ( 432.4999999999999432, 207.5000000000000284, 0.000000000000000000 ) ) ;
#62059=DIRECTION ( 'NONE',  ( 0.000000000000000000, 0.000000000000000000, -1.000000000000000000 ) ) ;
#62079=DIRECTION ( 'NONE',  ( 0.000000000000000000, 1.000000000000000000, 0.000000000000000000 ) ) ;
#62143=AXIS2_PLACEMENT_3D ( 'NONE', #18855, #50857, #52239 ) ;
#62168=AXIS2_PLACEMENT_3D ( 'NONE', #6291, #675, #59738 ) ;
#62190=ADVANCED_FACE ( 'NONE', ( #51854, #36370, #4018, #31105, #14570, #58170 ), #57829, .T. ) ;
#62205=DIRECTION ( 'NONE',  ( 0.000000000000000000, 0.000000000000000000, 1.000000000000000000 ) ) ;
#62233=VERTEX_POINT ( 'NONE', #67702 ) ;
#62237=AXIS2_PLACEMENT_3D ( 'NONE', #29108, #40346, #25568 ) ;
#62279=EDGE_CURVE ( 'NONE', #56653, #15171, #8665, .T. ) ;
#62283=AXIS2_PLACEMENT_3D ( 'NONE', #24844, #36783, #9349 ) ;
#62335=CIRCLE ( 'NONE', #58951, 5.000000000000004441 ) ;
#62341=CYLINDRICAL_SURFACE ( 'NONE', #28233, 245.3095347406802205 ) ;
#62375=ORIENTED_EDGE ( 'NONE', *, *, #64818, .F. ) ;
#62384=AXIS2_PLACEMENT_3D ( 'NONE', #13754, #13076, #67575 ) ;
#62386=CARTESIAN_POINT ( 'NONE',  ( 111.9975424824652634, 0.000000000000000000, 256.6193948016162381 ) ) ;
#62397=CARTESIAN_POINT ( 'NONE',  ( 141.9165763529819344, -2.000000000000001776, 129.0000000000000000 ) ) ;
#62401=CARTESIAN_POINT ( 'NONE',  ( 311.9975424824652350, 172.0000000000000000, 529.9060149868649887 ) ) ;
#62477=AXIS2_PLACEMENT_3D ( 'NONE', #61992, #3604, #25072 ) ;
#62505=FACE_BOUND ( 'NONE', #9586, .T. ) ;
#62509=EDGE_LOOP ( 'NONE', ( #22626, #59642, #41637, #7038 ) ) ;
#62523=AXIS2_PLACEMENT_3D ( 'NONE', #64954, #16750, #17088 ) ;
#62584=CARTESIAN_POINT ( 'NONE',  ( 444.9999999999999432, -35.00000000000000000, 380.0000000000000000 ) ) ;
#62591=EDGE_CURVE ( 'NONE', #47824, #18390, #39241, .T. ) ;
#62604=ORIENTED_EDGE ( 'NONE', *, *, #3498, .F. ) ;
#62619=ORIENTED_EDGE ( 'NONE', *, *, #50188, .F. ) ;
#62624=AXIS2_PLACEMENT_3D ( 'NONE', #16539, #27429, #48866 ) ;
#62631=CARTESIAN_POINT ( 'NONE',  ( 309.8720357909272707, 172.0000000000000284, 256.6193948016162381 ) ) ;
#62673=DIRECTION ( 'NONE',  ( 1.000000000000000000, 0.000000000000000000, -0.000000000000000000 ) ) ;
#62675=ORIENTED_EDGE ( 'NONE', *, *, #31931, .T. ) ;
#62679=VERTEX_POINT ( 'NONE', #29374 ) ;
#62690=ORIENTED_EDGE ( 'NONE', *, *, #21820, .F. ) ;
#62691=CARTESIAN_POINT ( 'NONE',  ( 266.9165763529819628, -2.000000000000001776, 128.9999999999999716 ) ) ;
#62715=ORIENTED_EDGE ( 'NONE', *, *, #20387, .T. ) ;
#62737=LINE ( 'NONE', #62386, #52566 ) ;
#62747=ORIENTED_EDGE ( 'NONE', *, *, #58511, .T. ) ;
#62775=DIRECTION ( 'NONE',  ( 0.008343357611898890094, 0.000000000000000000, 0.9999651935861366692 ) ) ;
#62812=MANIFOLD_SOLID_BREP ( 'Cut-Extrude7', #29416 ) ;
#62824=EDGE_CURVE ( 'NONE', #37937, #29599, #57493, .T. ) ;
#62862=ORIENTED_EDGE ( 'NONE', *, *, #30989, .F. ) ;
#62901=ORIENTED_EDGE ( 'NONE', *, *, #4527, .F. ) ;
#62945=CARTESIAN_POINT ( 'NONE',  ( -17.50000000000002842, -18.06806526123148160, 0.000000000000000000 ) ) ;
#62946=ORIENTED_EDGE ( 'NONE', *, *, #30021, .F. ) ;
#62952=DIRECTION ( 'NONE',  ( 1.000000000000000000, 0.000000000000000000, 0.000000000000000000 ) ) ;
#62987=CIRCLE ( 'NONE', #9119, 21.00000000000000355 ) ;
#62990=ORIENTED_EDGE ( 'NONE', *, *, #62824, .T. ) ;
#62998=EDGE_LOOP ( 'NONE', ( #56831, #39973, #43375, #57528, #57180, #12677, #52752, #66965, #23548 ) ) ;
#63033=AXIS2_PLACEMENT_3D ( 'NONE', #30059, #13863, #51513 ) ;
#63050=FACE_OUTER_BOUND ( 'NONE', #35079, .T. ) ;
#63055=ADVANCED_FACE ( 'NONE', ( #7838 ), #67291, .F. ) ;
#63082=CARTESIAN_POINT ( 'NONE',  ( 141.9165763529819344, -2.000000000000001776, 108.9999999999999858 ) ) ;
#63084=VECTOR ( 'NONE', #23726, 1000.000000000000000 ) ;
#63094=VERTEX_POINT ( 'NONE', #62691 ) ;
#63095=AXIS2_PLACEMENT_3D ( 'NONE', #29290, #50743, #24020 ) ;
#63112=SURFACE_STYLE_USAGE ( .BOTH. , #4026 ) ;
#63129=EDGE_CURVE ( 'NONE', #45635, #67175, #67178, .T. ) ;
#63191=VECTOR ( 'NONE', #69511, 1000.000000000000000 ) ;
#63193=LINE ( 'NONE', #30842, #10300 ) ;
#63219=ORIENTED_EDGE ( 'NONE', *, *, #59931, .T. ) ;
#63221=DIRECTION ( 'NONE',  ( -1.000000000000000000, 0.000000000000000000, 0.000000000000000000 ) ) ;
#63222=DIRECTION ( 'NONE',  ( 0.01527021686369653929, 0.000000000000000000, 0.9998834034410890581 ) ) ;
#63225=DIRECTION ( 'NONE',  ( -1.000000000000000000, 0.000000000000000000, 0.000000000000000000 ) ) ;
#63250=EDGE_CURVE ( 'NONE', #58728, #14130, #55228, .T. ) ;
#63311=CARTESIAN_POINT ( 'NONE',  ( -12.50000000000002842, -18.06806526123148160, 0.000000000000000000 ) ) ;
#63316=CARTESIAN_POINT ( 'NONE',  ( 444.9999999999999432, 225.0000000000000000, -2.000000000000000000 ) ) ;
#63358=ORIENTED_EDGE ( 'NONE', *, *, #56442, .T. ) ;
#63360=FACE_OUTER_BOUND ( 'NONE', #45690, .T. ) ;
#63362=ORIENTED_EDGE ( 'NONE', *, *, #43981, .T. ) ;
#63369=EDGE_LOOP ( 'NONE', ( #21266, #65176, #39034, #29142 ) ) ;
#63399=ORIENTED_EDGE ( 'NONE', *, *, #18623, .F. ) ;
#63404=CARTESIAN_POINT ( 'NONE',  ( -17.50000000000002842, 207.5000000000000284, 0.000000000000000000 ) ) ;
#63442=VECTOR ( 'NONE', #68470, 1000.000000000000000 ) ;
#63473=DIRECTION ( 'NONE',  ( -1.000000000000000000, 0.000000000000000000, -0.000000000000000000 ) ) ;
#63491=ORIENTED_EDGE ( 'NONE', *, *, #67416, .F. ) ;
#63527=ORIENTED_EDGE ( 'NONE', *, *, #27801, .F. ) ;
#63551=ADVANCED_FACE ( 'NONE', ( #19168 ), #34328, .F. ) ;
#63611=ADVANCED_FACE ( 'NONE', ( #35011, #8635, #56456 ), #8284, .F. ) ;
#63631=CARTESIAN_POINT ( 'NONE',  ( 209.9518228411288874, 20.00000000000003197, 31.43423095485942298 ) ) ;
#63632=VECTOR ( 'NONE', #9788, 1000.000000000000000 ) ;
#63649=LINE ( 'NONE', #57330, #14335 ) ;
#63686=VECTOR ( 'NONE', #50804, 1000.000000000000000 ) ;
#63758=CARTESIAN_POINT ( 'NONE',  ( 149.4165763529819344, -26.99999999999998224, 129.0000000000000000 ) ) ;
#63825=ORIENTED_EDGE ( 'NONE', *, *, #7578, .F. ) ;
#63840=CIRCLE ( 'NONE', #25649, 5.000000000000004441 ) ;
#63881=DIRECTION ( 'NONE',  ( 0.000000000000000000, -0.1086713087885527451, -0.9940777367219241212 ) ) ;
#63904=DIRECTION ( 'NONE',  ( 0.000000000000000000, 0.000000000000000000, -1.000000000000000000 ) ) ;
#63905=DIRECTION ( 'NONE',  ( 0.000000000000000000, -0.000000000000000000, -1.000000000000000000 ) ) ;
#63925=EDGE_CURVE ( 'NONE', #22108, #36497, #2086, .T. ) ;
#63936=LINE ( 'NONE', #15747, #63632 ) ;
#64007=VECTOR ( 'NONE', #64416, 1000.000000000000000 ) ;
#64022=EDGE_CURVE ( 'NONE', #14720, #59570, #42859, .T. ) ;
#64024=AXIS2_PLACEMENT_3D ( 'NONE', #40513, #41212, #62673 ) ;
#64068=DIRECTION ( 'NONE',  ( 0.000000000000000000, 1.000000000000000000, -0.000000000000000000 ) ) ;
#64091=DIRECTION ( 'NONE',  ( 2.220446049250313081E-16, 0.000000000000000000, 1.000000000000000000 ) ) ;
#64098=CARTESIAN_POINT ( 'NONE',  ( -17.50000000000002842, -18.06806526123148160, 0.000000000000000000 ) ) ;
#64109=CARTESIAN_POINT ( 'NONE',  ( -17.50000000000002842, -18.06806526123148160, 378.0000000000000000 ) ) ;
#64128=FACE_OUTER_BOUND ( 'NONE', #32939, .T. ) ;
#64140=SURFACE_STYLE_FILL_AREA ( #52209 ) ;
#64162=EDGE_CURVE ( 'NONE', #35195, #60279, #1708, .T. ) ;
#64182=CIRCLE ( 'NONE', #13688, 21.00000000000000355 ) ;
#64214=ADVANCED_FACE ( 'NONE', ( #55156 ), #6980, .T. ) ;
#64300=DIRECTION ( 'NONE',  ( 0.000000000000000000, 1.000000000000000000, -0.000000000000000000 ) ) ;
#64359=DIRECTION ( 'NONE',  ( 1.000000000000000000, 0.000000000000000000, 0.000000000000000000 ) ) ;
#64374=PLANE ( 'NONE',  #49964 ) ;
#64392=DIRECTION ( 'NONE',  ( -0.000000000000000000, 1.000000000000000000, -0.000000000000000000 ) ) ;
#64394=ORIENTED_EDGE ( 'NONE', *, *, #10636, .T. ) ;
#64416=DIRECTION ( 'NONE',  ( 0.000000000000000000, 1.000000000000000000, 0.000000000000000000 ) ) ;
#64435=CARTESIAN_POINT ( 'NONE',  ( 444.9999999999999432, 225.0000000000000000, 380.0000000000000000 ) ) ;
#64442=AXIS2_PLACEMENT_3D ( 'NONE', #2119, #49579, #13022 ) ;
#64444=CARTESIAN_POINT ( 'NONE',  ( 230.9999999999999432, -57.00000000000007816, 72.99999999999998579 ) ) ;
#64509=DIRECTION ( 'NONE',  ( -1.000000000000000000, 0.000000000000000000, 0.000000000000000000 ) ) ;
#64526=DIRECTION ( 'NONE',  ( -0.000000000000000000, -0.000000000000000000, 1.000000000000000000 ) ) ;
#64554=DIRECTION ( 'NONE',  ( 0.000000000000000000, 1.000000000000000000, 0.000000000000000000 ) ) ;
#64588=VECTOR ( 'NONE', #67026, 1000.000000000000000 ) ;
#64614=LINE ( 'NONE', #15736, #51337 ) ;
#64628=LINE ( 'NONE', #17835, #35617 ) ;
#64631=EDGE_CURVE ( 'NONE', #59483, #60423, #12570, .T. ) ;
#64644=CARTESIAN_POINT ( 'NONE',  ( 111.9975424824652634, 296.0000000000000000, 420.0000000000000568 ) ) ;
#64729=DIRECTION ( 'NONE',  ( 0.000000000000000000, -0.9989683093773507050, -0.04541273895899305274 ) ) ;
#64791=ORIENTED_EDGE ( 'NONE', *, *, #42105, .F. ) ;
#64799=DIRECTION ( 'NONE',  ( -0.000000000000000000, -0.000000000000000000, -1.000000000000000000 ) ) ;
#64812=DIRECTION ( 'NONE',  ( -0.000000000000000000, -0.000000000000000000, -1.000000000000000000 ) ) ;
#64814=DIRECTION ( 'NONE',  ( -0.000000000000000000, -1.000000000000000000, 0.000000000000000000 ) ) ;
#64817=EDGE_CURVE ( 'NONE', #52456, #35904, #8958, .T. ) ;
#64818=EDGE_CURVE ( 'NONE', #40730, #41180, #21634, .T. ) ;
#64830=AXIS2_PLACEMENT_3D ( 'NONE', #40403, #2097, #62205 ) ;
#64845=FACE_OUTER_BOUND ( 'NONE', #23773, .T. ) ;
#64867=VECTOR ( 'NONE', #3156, 1000.000000000000000 ) ;
#64935=AXIS2_PLACEMENT_3D ( 'NONE', #29729, #51194, #69068 ) ;
#64939=LINE ( 'NONE', #31292, #24224 ) ;
#64954=CARTESIAN_POINT ( 'NONE',  ( 427.4999999999999432, 207.5000000000000284, -2.000000000000000000 ) ) ;
#64965=EDGE_CURVE ( 'NONE', #45190, #41448, #12139, .T. ) ;
#64968=CARTESIAN_POINT ( 'NONE',  ( 141.9165763529819344, -52.00000000000000711, 108.9999999999999858 ) ) ;
#64989=CARTESIAN_POINT ( 'NONE',  ( 230.9999999999999432, -57.00000000000007816, 72.99999999999998579 ) ) ;
#65005=VERTEX_POINT ( 'NONE', #62048 ) ;
#65014=CARTESIAN_POINT ( 'NONE',  ( -22.50000000000003197, -18.06806526123148160, 0.000000000000000000 ) ) ;
#65026=ORIENTED_EDGE ( 'NONE', *, *, #53401, .T. ) ;
#65062=ORIENTED_EDGE ( 'NONE', *, *, #41069, .F. ) ;
#65083=ORIENTED_EDGE ( 'NONE', *, *, #473, .F. ) ;
#65085=LINE ( 'NONE', #53735, #50850 ) ;
#65106=CARTESIAN_POINT ( 'NONE',  ( 109.9975424824652634, 18.08738615523480675, 402.4289050101931480 ) ) ;
#65126=LINE ( 'NONE', #16922, #67775 ) ;
#65176=ORIENTED_EDGE ( 'NONE', *, *, #55743, .F. ) ;
#65188=DIRECTION ( 'NONE',  ( -0.000000000000000000, -0.000000000000000000, -1.000000000000000000 ) ) ;
#65192=ORIENTED_EDGE ( 'NONE', *, *, #60489, .T. ) ;
#65220=ORIENTED_EDGE ( 'NONE', *, *, #27041, .F. ) ;
#65242=CARTESIAN_POINT ( 'NONE',  ( 422.4999999999999432, -18.06806526123148160, 0.000000000000000000 ) ) ;
#65244=ORIENTED_EDGE ( 'NONE', *, *, #51181, .T. ) ;
#65247=EDGE_LOOP ( 'NONE', ( #19297, #7026, #63219, #58176 ) ) ;
#65250=ORIENTED_EDGE ( 'NONE', *, *, #32094, .T. ) ;
#65287=ORIENTED_EDGE ( 'NONE', *, *, #39463, .F. ) ;
#65338=CARTESIAN_POINT ( 'NONE',  ( 211.9972138934681425, 190.0000000000000000, 276.7374251518728556 ) ) ;
#65339=LINE ( 'NONE', #7652, #58501 ) ;
#65343=ORIENTED_EDGE ( 'NONE', *, *, #4439, .T. ) ;
#65367=CARTESIAN_POINT ( 'NONE',  ( 209.3223706822284100, 18.00000000000002842, 31.44247402469554942 ) ) ;
#65376=ORIENTED_EDGE ( 'NONE', *, *, #53398, .T. ) ;
#65386=CYLINDRICAL_SURFACE ( 'NONE', #60645, 5.000000000000000888 ) ;
#65400=LINE ( 'NONE', #66460, #13145 ) ;
#65412=ORIENTED_EDGE ( 'NONE', *, *, #58675, .T. ) ;
#65428=DIRECTION ( 'NONE',  ( 0.000000000000000000, -0.04541273895899305968, 0.9989683093773508160 ) ) ;
#65435=DIRECTION ( 'NONE',  ( 0.000000000000000000, 0.000000000000000000, 1.000000000000000000 ) ) ;
#65442=ADVANCED_FACE ( 'NONE', ( #29272 ), #39823, .F. ) ;
#65443=AXIS2_PLACEMENT_3D ( 'NONE', #1413, #39398, #23915 ) ;
#65444=VERTEX_POINT ( 'NONE', #23997 ) ;
#65449=ORIENTED_EDGE ( 'NONE', *, *, #1558, .T. ) ;
#65471=ADVANCED_FACE ( 'NONE', ( #45443, #14131, #29967 ), #29608, .F. ) ;
#65503=LINE ( 'NONE', #48590, #360 ) ;
#65518=DIRECTION ( 'NONE',  ( -0.000000000000000000, -0.000000000000000000, -1.000000000000000000 ) ) ;
#65521=ORIENTED_EDGE ( 'NONE', *, *, #21196, .T. ) ;
#65546=ORIENTED_EDGE ( 'NONE', *, *, #2654, .F. ) ;
#65569=DIRECTION ( 'NONE',  ( 2.220446049250313081E-16, -0.000000000000000000, 1.000000000000000000 ) ) ;
#65652=DIRECTION ( 'NONE',  ( 0.000000000000000000, 0.000000000000000000, 1.000000000000000000 ) ) ;
#65661=VERTEX_POINT ( 'NONE', #43526 ) ;
#65676=ORIENTED_EDGE ( 'NONE', *, *, #51091, .T. ) ;
#65699=LINE ( 'NONE', #60047, #13371 ) ;
#65731=ORIENTED_EDGE ( 'NONE', *, *, #56960, .F. ) ;
#65753=CARTESIAN_POINT ( 'NONE',  ( 188.9999999999999432, 0.000000000000000000, -2.000000000000000888 ) ) ;
#65773=EDGE_CURVE ( 'NONE', #30991, #69498, #60759, .T. ) ;
#65838=ORIENTED_EDGE ( 'NONE', *, *, #14536, .T. ) ;
#65851=DIRECTION ( 'NONE',  ( 1.000000000000000000, 0.000000000000000000, 0.000000000000000000 ) ) ;
#65860=CARTESIAN_POINT ( 'NONE',  ( 254.4165763529819344, -27.00000000000000355, 108.9999999999999858 ) ) ;
#65878=DIRECTION ( 'NONE',  ( -1.000000000000000000, 0.000000000000000000, 2.775557561562891844E-16 ) ) ;
#65888=DIRECTION ( 'NONE',  ( -2.220446049250313081E-16, 0.000000000000000000, -1.000000000000000000 ) ) ;
#65941=ORIENTED_EDGE ( 'NONE', *, *, #27801, .T. ) ;
#65946=EDGE_CURVE ( 'NONE', #44768, #28503, #48357, .T. ) ;
#65970=DIRECTION ( 'NONE',  ( 0.000000000000000000, 1.000000000000000000, 0.000000000000000000 ) ) ;
#65985=EDGE_LOOP ( 'NONE', ( #53755, #5814, #10893, #48302 ) ) ;
#66006=LINE ( 'NONE', #33291, #30668 ) ;
#66034=CARTESIAN_POINT ( 'NONE',  ( -22.50000000000003197, 207.5000000000000284, 378.0000000000000000 ) ) ;
#66091=ADVANCED_FACE ( 'NONE', ( #55045 ), #27971, .F. ) ;
#66107=ORIENTED_EDGE ( 'NONE', *, *, #29230, .T. ) ;
#66110=LINE ( 'NONE', #8394, #68114 ) ;
#66147=FACE_BOUND ( 'NONE', #10937, .T. ) ;
#66152=VERTEX_POINT ( 'NONE', #29037 ) ;
#66164=AXIS2_PLACEMENT_3D ( 'NONE', #45745, #61906, #4899 ) ;
#66167=CARTESIAN_POINT ( 'NONE',  ( 410.0000000000000000, 190.0000000000000000, -2.000000000000000000 ) ) ;
#66171=CARTESIAN_POINT ( 'NONE',  ( 0.000000000000000000, 0.000000000000000000, 380.0000000000000000 ) ) ;
#66177=EDGE_LOOP ( 'NONE', ( #31230, #54653 ) ) ;
#66188=DIRECTION ( 'NONE',  ( -1.000000000000000000, 0.000000000000000000, 0.000000000000000000 ) ) ;
#66198=CARTESIAN_POINT ( 'NONE',  ( 309.8720357909272707, 18.00000000000002842, 256.6193948016162381 ) ) ;
#66209=ORIENTED_EDGE ( 'NONE', *, *, #65773, .F. ) ;
#66218=ORIENTED_EDGE ( 'NONE', *, *, #48424, .T. ) ;
#66276=CARTESIAN_POINT ( 'NONE',  ( 188.9999999999999432, -57.00000000000007816, 72.99999999999998579 ) ) ;
#66300=DIRECTION ( 'NONE',  ( -0.000000000000000000, -0.000000000000000000, -1.000000000000000000 ) ) ;
#66322=EDGE_CURVE ( 'NONE', #5206, #40354, #7902, .T. ) ;
#66324=EDGE_LOOP ( 'NONE', ( #42566, #696, #40005, #53459 ) ) ;
#66329=CARTESIAN_POINT ( 'NONE',  ( 0.000000000000000000, 0.000000000000000000, 380.0000000000000000 ) ) ;
#66333=CARTESIAN_POINT ( 'NONE',  ( 313.9975424824652350, 307.8795515535290974, 6.994434899193393562 ) ) ;
#66354=CARTESIAN_POINT ( 'NONE',  ( 309.8720357909272707, 172.0000000000000284, 256.6193948016162381 ) ) ;
#66374=DIRECTION ( 'NONE',  ( 0.000000000000000000, -0.000000000000000000, 1.000000000000000000 ) ) ;
#66408=EDGE_CURVE ( 'NONE', #16482, #55258, #59883, .T. ) ;
#66433=CARTESIAN_POINT ( 'NONE',  ( -2.000000000000000000, -2.000000000000000000, 378.0000000000000000 ) ) ;
#66438=CARTESIAN_POINT ( 'NONE',  ( 313.9975424824652350, 296.0000000000000000, 418.0000000000000000 ) ) ;
#66456=PLANE ( 'NONE',  #19207 ) ;
#66460=CARTESIAN_POINT ( 'NONE',  ( 111.9975424824652634, 20.00000000000003197, 401.6295345748407613 ) ) ;
#66461=EDGE_LOOP ( 'NONE', ( #45453, #66209, #59137, #65449 ) ) ;
#66484=AXIS2_PLACEMENT_3D ( 'NONE', #27987, #50149, #60351 ) ;
#66499=ORIENTED_EDGE ( 'NONE', *, *, #24472, .T. ) ;
#66505=CARTESIAN_POINT ( 'NONE',  ( 444.9999999999999432, -35.00000000000000000, 0.000000000000000000 ) ) ;
#66561=DIRECTION ( 'NONE',  ( 1.000000000000000000, -0.000000000000000000, 0.000000000000000000 ) ) ;
#66569=AXIS2_PLACEMENT_3D ( 'NONE', #46303, #14991, #3750 ) ;
#66577=CARTESIAN_POINT ( 'NONE',  ( 149.4165763529819344, 225.8585178651493663, 138.9999999999999716 ) ) ;
#66591=EDGE_CURVE ( 'NONE', #18335, #56454, #48196, .T. ) ;
#66625=ORIENTED_EDGE ( 'NONE', *, *, #1020, .T. ) ;
#66661=ORIENTED_EDGE ( 'NONE', *, *, #58572, .T. ) ;
#66671=AXIS2_PLACEMENT_3D ( 'NONE', #3278, #7251, #19797 ) ;
#66680=VECTOR ( 'NONE', #17118, 1000.000000000000000 ) ;
#66692=DIRECTION ( 'NONE',  ( 1.000000000000000000, 0.000000000000000000, 0.000000000000000000 ) ) ;
#66693=CARTESIAN_POINT ( 'NONE',  ( 209.3223706822284100, 0.000000000000000000, 276.7520087653757628 ) ) ;
#66702=CARTESIAN_POINT ( 'NONE',  ( 309.8720357909272707, 18.00000000000002842, 536.6193948016162949 ) ) ;
#66713=EDGE_CURVE ( 'NONE', #67398, #17316, #8088, .T. ) ;
#66738=EDGE_CURVE ( 'NONE', #69500, #52338, #67884, .T. ) ;
#66756=CARTESIAN_POINT ( 'NONE',  ( 266.9165763529819628, -52.00000000000000711, 108.9999999999999858 ) ) ;
#66758=VERTEX_POINT ( 'NONE', #3169 ) ;
#66798=ORIENTED_EDGE ( 'NONE', *, *, #32481, .T. ) ;
#66809=ORIENTED_EDGE ( 'NONE', *, *, #37677, .F. ) ;
#66815=DIRECTION ( 'NONE',  ( 0.000000000000000000, 0.000000000000000000, -1.000000000000000000 ) ) ;
#66823=ADVANCED_FACE ( 'NONE', ( #40443 ), #2816, .F. ) ;
#66827=LINE ( 'NONE', #22847, #42478 ) ;
#66829=VECTOR ( 'NONE', #35311, 1000.000000000000000 ) ;
#66832=AXIS2_PLACEMENT_3D ( 'NONE', #50530, #44558, #8319 ) ;
#66836=DIRECTION ( 'NONE',  ( 1.000000000000000000, 0.000000000000000000, 0.000000000000000000 ) ) ;
#66844=DIRECTION ( 'NONE',  ( 0.000000000000000000, 0.000000000000000000, -1.000000000000000000 ) ) ;
#66847=DIRECTION ( 'NONE',  ( 1.000000000000000000, 0.000000000000000000, 0.000000000000000000 ) ) ;
#66851=ORIENTED_EDGE ( 'NONE', *, *, #21265, .T. ) ;
#66856=EDGE_LOOP ( 'NONE', ( #52086, #62619 ) ) ;
#66898=ORIENTED_EDGE ( 'NONE', *, *, #45038, .F. ) ;
#66949=VERTEX_POINT ( 'NONE', #10157 ) ;
#66965=ORIENTED_EDGE ( 'NONE', *, *, #20529, .T. ) ;
#66966=PLANE ( 'NONE',  #59037 ) ;
#66973=CIRCLE ( 'NONE', #42244, 5.000000000000000888 ) ;
#67014=CARTESIAN_POINT ( 'NONE',  ( 109.9975424824652777, 296.0000000000000000, 418.0000000000000000 ) ) ;
#67018=FACE_OUTER_BOUND ( 'NONE', #3790, .T. ) ;
#67026=DIRECTION ( 'NONE',  ( 1.000000000000000000, 0.000000000000000000, -0.000000000000000000 ) ) ;
#67054=EDGE_CURVE ( 'NONE', #7837, #66152, #51901, .T. ) ;
#67110=VECTOR ( 'NONE', #57379, 1000.000000000000000 ) ;
#67150=CARTESIAN_POINT ( 'NONE',  ( 209.9999999999999716, 0.000000000000000000, 72.99999999999998579 ) ) ;
#67153=DIRECTION ( 'NONE',  ( 0.000000000000000000, -1.000000000000000000, 0.000000000000000000 ) ) ;
#67175=VERTEX_POINT ( 'NONE', #65014 ) ;
#67178=CIRCLE ( 'NONE', #13232, 5.000000000000000888 ) ;
#67191=LINE ( 'NONE', #46050, #61137 ) ;
#67203=DIRECTION ( 'NONE',  ( 0.000000000000000000, 1.000000000000000000, 0.000000000000000000 ) ) ;
#67204=DIRECTION ( 'NONE',  ( -1.000000000000000000, 0.000000000000000000, 0.000000000000000000 ) ) ;
#67211=CARTESIAN_POINT ( 'NONE',  ( 209.3223706822284100, 172.0000000000000284, 31.44247402469554942 ) ) ;
#67254=ORIENTED_EDGE ( 'NONE', *, *, #58667, .F. ) ;
#67279=ORIENTED_EDGE ( 'NONE', *, *, #54648, .F. ) ;
#67283=LINE ( 'NONE', #29617, #25780 ) ;
#67291=CYLINDRICAL_SURFACE ( 'NONE', #26675, 21.00000000000000355 ) ;
#67311=VERTEX_POINT ( 'NONE', #39670 ) ;
#67314=VECTOR ( 'NONE', #27890, 1000.000000000000000 ) ;
#67336=CARTESIAN_POINT ( 'NONE',  ( 410.0000000000000000, 190.0000000000000000, 380.0000000000000000 ) ) ;
#67351=EDGE_CURVE ( 'NONE', #60423, #54755, #55397, .T. ) ;
#67358=PLANE ( 'NONE',  #8753 ) ;
#67359=VECTOR ( 'NONE', #16981, 1000.000000000000000 ) ;
#67398=VERTEX_POINT ( 'NONE', #26858 ) ;
#67416=EDGE_CURVE ( 'NONE', #15171, #5460, #38096, .T. ) ;
#67514=EDGE_CURVE ( 'NONE', #55844, #41662, #65126, .T. ) ;
#67520=DIRECTION ( 'NONE',  ( 0.000000000000000000, 1.000000000000000000, 0.000000000000000000 ) ) ;
#67534=EDGE_CURVE ( 'NONE', #26255, #28668, #21704, .T. ) ;
#67537=ORIENTED_EDGE ( 'NONE', *, *, #18444, .F. ) ;
#67575=DIRECTION ( 'NONE',  ( 0.000000000000000000, -0.000000000000000000, 1.000000000000000000 ) ) ;
#67578=CARTESIAN_POINT ( 'NONE',  ( 141.9165763529819344, 192.0000000000000000, 108.9999999999999289 ) ) ;
#67626=CARTESIAN_POINT ( 'NONE',  ( 422.4999999999999432, 207.5000000000000284, 378.0000000000000000 ) ) ;
#67686=AXIS2_PLACEMENT_3D ( 'NONE', #16465, #61116, #18208 ) ;
#67702=CARTESIAN_POINT ( 'NONE',  ( 311.9975424824652350, 172.0000000000000284, 420.0000000000000568 ) ) ;
#67721=DIRECTION ( 'NONE',  ( 1.000000000000000000, 0.000000000000000000, -0.000000000000000000 ) ) ;
#67732=CARTESIAN_POINT ( 'NONE',  ( 412.0000000000000000, 0.000000000000000000, 380.0000000000000000 ) ) ;
#67736=CARTESIAN_POINT ( 'NONE',  ( 259.4165763529819060, 225.8585178651493948, 138.9999999999999716 ) ) ;
#67738=DIRECTION ( 'NONE',  ( -1.000000000000000000, 0.000000000000000000, 0.000000000000000000 ) ) ;
#67741=EDGE_LOOP ( 'NONE', ( #27645, #1496 ) ) ;
#67747=CARTESIAN_POINT ( 'NONE',  ( 444.9999999999999432, 225.0000000000000000, 378.0000000000000000 ) ) ;
#67775=VECTOR ( 'NONE', #38386, 1000.000000000000000 ) ;
#67787=DIRECTION ( 'NONE',  ( 0.000000000000000000, 0.000000000000000000, -1.000000000000000000 ) ) ;
#67792=ORIENTED_EDGE ( 'NONE', *, *, #50417, .F. ) ;
#67823=ADVANCED_FACE ( 'NONE', ( #25002 ), #41172, .T. ) ;
#67836=EDGE_CURVE ( 'NONE', #44768, #39465, #36238, .T. ) ;
#67846=CARTESIAN_POINT ( 'NONE',  ( 254.4165763529819344, 225.8585178651493948, 138.9999999999999716 ) ) ;
#67884=LINE ( 'NONE', #66505, #49626 ) ;
#67887=ADVANCED_FACE ( 'NONE', ( #43909 ), #48474, .F. ) ;
#67891=DIRECTION ( 'NONE',  ( -0.000000000000000000, -0.000000000000000000, -1.000000000000000000 ) ) ;
#67911=ORIENTED_EDGE ( 'NONE', *, *, #44720, .T. ) ;
#67912=AXIS2_PLACEMENT_3D ( 'NONE', #56898, #29119, #8365 ) ;
#67937=EDGE_CURVE ( 'NONE', #33294, #26166, #48144, .T. ) ;
#67950=CARTESIAN_POINT ( 'NONE',  ( 309.8720357909272707, 172.0000000000000284, 256.6193948016162381 ) ) ;
#68005=DIRECTION ( 'NONE',  ( 0.000000000000000000, -1.000000000000000000, 0.000000000000000000 ) ) ;
#68048=DIRECTION ( 'NONE',  ( 1.000000000000000000, 0.000000000000000000, 0.000000000000000000 ) ) ;
#68055=CARTESIAN_POINT ( 'NONE',  ( 111.9975424824652634, 172.0000000000002274, 529.9060149868648750 ) ) ;
#68068=VERTEX_POINT ( 'NONE', #6639 ) ;
#68072=CARTESIAN_POINT ( 'NONE',  ( -2.000000000000000000, 0.000000000000000000, 380.0000000000000000 ) ) ;
#68093=ORIENTED_EDGE ( 'NONE', *, *, #69395, .F. ) ;
#68095=LINE ( 'NONE', #31483, #49859 ) ;
#68103=SHAPE_REPRESENTATION_RELATIONSHIP ( 'NONE' , 'NONE' ,  #57739, #55050 ) ;
#68114=VECTOR ( 'NONE', #67153, 1000.000000000000000 ) ;
#68136=EDGE_CURVE ( 'NONE', #56285, #22108, #6030, .T. ) ;
#68167=LINE ( 'NONE', #1812, #46651 ) ;
#68169=PRODUCT_DEFINITION_FORMATION_WITH_SPECIFIED_SOURCE ( 'ANY', '', #34472, .NOT_KNOWN. ) ;
#68185=CARTESIAN_POINT ( 'NONE',  ( 0.000000000000000000, -2.000000000000000000, -0.000000000000000000 ) ) ;
#68233=DIRECTION ( 'NONE',  ( 0.000000000000000000, -1.000000000000000000, -0.000000000000000000 ) ) ;
#68234=ORIENTED_EDGE ( 'NONE', *, *, #28849, .T. ) ;
#68240=EDGE_CURVE ( 'NONE', #1408, #13211, #44892, .T. ) ;
#68257=DIRECTION ( 'NONE',  ( 0.000000000000000000, 0.000000000000000000, -1.000000000000000000 ) ) ;
#68262=CARTESIAN_POINT ( 'NONE',  ( 230.9999999999999432, -2.000000000000000000, 380.0000000000000000 ) ) ;
#68264=MECHANICAL_DESIGN_GEOMETRIC_PRESENTATION_REPRESENTATION('',(#44660),#15482);
#68270=ORIENTED_EDGE ( 'NONE', *, *, #44479, .T. ) ;
#68283=EDGE_CURVE ( 'NONE', #11879, #54755, #45584, .T. ) ;
#68297=ADVANCED_FACE ( 'NONE', ( #44176 ), #12897, .T. ) ;
#68320=DIRECTION ( 'NONE',  ( 0.000000000000000000, 0.000000000000000000, -1.000000000000000000 ) ) ;
#68322=ADVANCED_FACE ( 'NONE', ( #50170 ), #18167, .F. ) ;
#68381=EDGE_LOOP ( 'NONE', ( #19984, #19758, #54507, #27983 ) ) ;
#68440=DIRECTION ( 'NONE',  ( 1.000000000000000000, 0.000000000000000000, -2.775557561562891844E-16 ) ) ;
#68470=DIRECTION ( 'NONE',  ( -0.000000000000000000, 1.000000000000000000, -0.000000000000000000 ) ) ;
#68495=LINE ( 'NONE', #20300, #8215 ) ;
#68503=VERTEX_POINT ( 'NONE', #53170 ) ;
#68511=CARTESIAN_POINT ( 'NONE',  ( 188.9999999999999432, -57.00000000000007816, -2.000000000000000888 ) ) ;
#68515=EDGE_CURVE ( 'NONE', #2626, #50048, #43132, .T. ) ;
#68575=EDGE_LOOP ( 'NONE', ( #54091, #6535, #34120, #50121 ) ) ;
#68577=ORIENTED_EDGE ( 'NONE', *, *, #49365, .T. ) ;
#68603=CARTESIAN_POINT ( 'NONE',  ( 209.3223706822284100, 18.00000000000002842, 31.44247402469554942 ) ) ;
#68623=CARTESIAN_POINT ( 'NONE',  ( 311.9975424824652350, 296.0000000000000000, 529.9060149868646477 ) ) ;
#68628=CYLINDRICAL_SURFACE ( 'NONE', #51841, 5.000000000000004441 ) ;
#68638=ORIENTED_EDGE ( 'NONE', *, *, #25425, .F. ) ;
#68666=VERTEX_POINT ( 'NONE', #1118 ) ;
#68704=AXIS2_PLACEMENT_3D ( 'NONE', #32822, #7497, #54610 ) ;
#68708=AXIS2_PLACEMENT_3D ( 'NONE', #5921, #11543, #28083 ) ;
#68742=DIRECTION ( 'NONE',  ( -0.000000000000000000, -0.000000000000000000, -1.000000000000000000 ) ) ;
#68769=PLANE ( 'NONE',  #24143 ) ;
#68778=ADVANCED_FACE ( 'NONE', ( #49992 ), #18332, .F. ) ;
#68787=VERTEX_POINT ( 'NONE', #7447 ) ;
#68791=DIRECTION ( 'NONE',  ( 0.000000000000000000, 1.000000000000000000, 0.000000000000000000 ) ) ;
#68837=DIRECTION ( 'NONE',  ( -1.000000000000000000, 0.000000000000000000, 0.000000000000000000 ) ) ;
#68845=ORIENTED_EDGE ( 'NONE', *, *, #3843, .T. ) ;
#68906=VECTOR ( 'NONE', #59318, 1000.000000000000000 ) ;
#68920=EDGE_CURVE ( 'NONE', #22014, #56285, #68929, .T. ) ;
#68929=LINE ( 'NONE', #20753, #13982 ) ;
#68949=AXIS2_PLACEMENT_3D ( 'NONE', #24616, #57655, #66844 ) ;
#68951=EDGE_LOOP ( 'NONE', ( #27703, #16417, #26920, #25895, #56302, #29163, #28197, #39959, #59204, #55955, #491, #57450 ) ) ;
#69004=EDGE_CURVE ( 'NONE', #68787, #67311, #27402, .T. ) ;
#69017=PLANE ( 'NONE',  #35266 ) ;
#69031=DIRECTION ( 'NONE',  ( 0.000000000000000000, 0.000000000000000000, -1.000000000000000000 ) ) ;
#69044=ORIENTED_EDGE ( 'NONE', *, *, #60985, .F. ) ;
#69050=CARTESIAN_POINT ( 'NONE',  ( 0.000000000000000000, 0.000000000000000000, 378.0000000000000000 ) ) ;
#69053=DIRECTION ( 'NONE',  ( -1.000000000000000000, 0.000000000000000000, 0.000000000000000000 ) ) ;
#69068=DIRECTION ( 'NONE',  ( 1.000000000000000000, 0.000000000000000000, -0.000000000000000000 ) ) ;
#69098=AXIS2_PLACEMENT_3D ( 'NONE', #7936, #23769, #61735 ) ;
#69125=ORIENTED_EDGE ( 'NONE', *, *, #297, .T. ) ;
#69128=VERTEX_POINT ( 'NONE', #1033 ) ;
#69137=LINE ( 'NONE', #47334, #16234 ) ;
#69148=EDGE_CURVE ( 'NONE', #59809, #68503, #23192, .T. ) ;
#69161=ORIENTED_EDGE ( 'NONE', *, *, #8569, .F. ) ;
#69175=DIRECTION ( 'NONE',  ( 0.000000000000000000, 0.000000000000000000, -1.000000000000000000 ) ) ;
#69182=ORIENTED_EDGE ( 'NONE', *, *, #3333, .T. ) ;
#69240=ORIENTED_EDGE ( 'NONE', *, *, #44865, .F. ) ;
#69243=EDGE_CURVE ( 'NONE', #48350, #25214, #39839, .T. ) ;
#69268=CARTESIAN_POINT ( 'NONE',  ( 313.9975424824652350, 295.6904194069557548, 539.5330678552892323 ) ) ;
#69302=FACE_BOUND ( 'NONE', #30784, .T. ) ;
#69317=ORIENTED_EDGE ( 'NONE', *, *, #38668, .T. ) ;
#69340=DIRECTION ( 'NONE',  ( 0.000000000000000000, 1.000000000000000000, 0.000000000000000000 ) ) ;
#69361=VERTEX_POINT ( 'NONE', #3463 ) ;
#69366=LINE ( 'NONE', #20833, #265 ) ;
#69390=EDGE_CURVE ( 'NONE', #32243, #28546, #21023, .T. ) ;
#69395=EDGE_CURVE ( 'NONE', #36317, #39465, #27318, .T. ) ;
#69396=CARTESIAN_POINT ( 'NONE',  ( 409.0783954480986608, -1.426547569622074412E-15, 174.7010307253933377 ) ) ;
#69411=VERTEX_POINT ( 'NONE', #10803 ) ;
#69450=VERTEX_POINT ( 'NONE', #26645 ) ;
#69498=VERTEX_POINT ( 'NONE', #37889 ) ;
#69500=VERTEX_POINT ( 'NONE', #15740 ) ;
#69511=DIRECTION ( 'NONE',  ( -0.000000000000000000, -1.000000000000000000, -0.000000000000000000 ) ) ;
#69533=CARTESIAN_POINT ( 'NONE',  ( 111.9975424824652634, 22.00669820036272384, 401.6295345748407613 ) ) ;
#69560=CARTESIAN_POINT ( 'NONE',  ( 141.9165763529819344, 192.0000000000000000, 129.0000000000000000 ) ) ;
ENDSEC;
END-ISO-10303-21;
